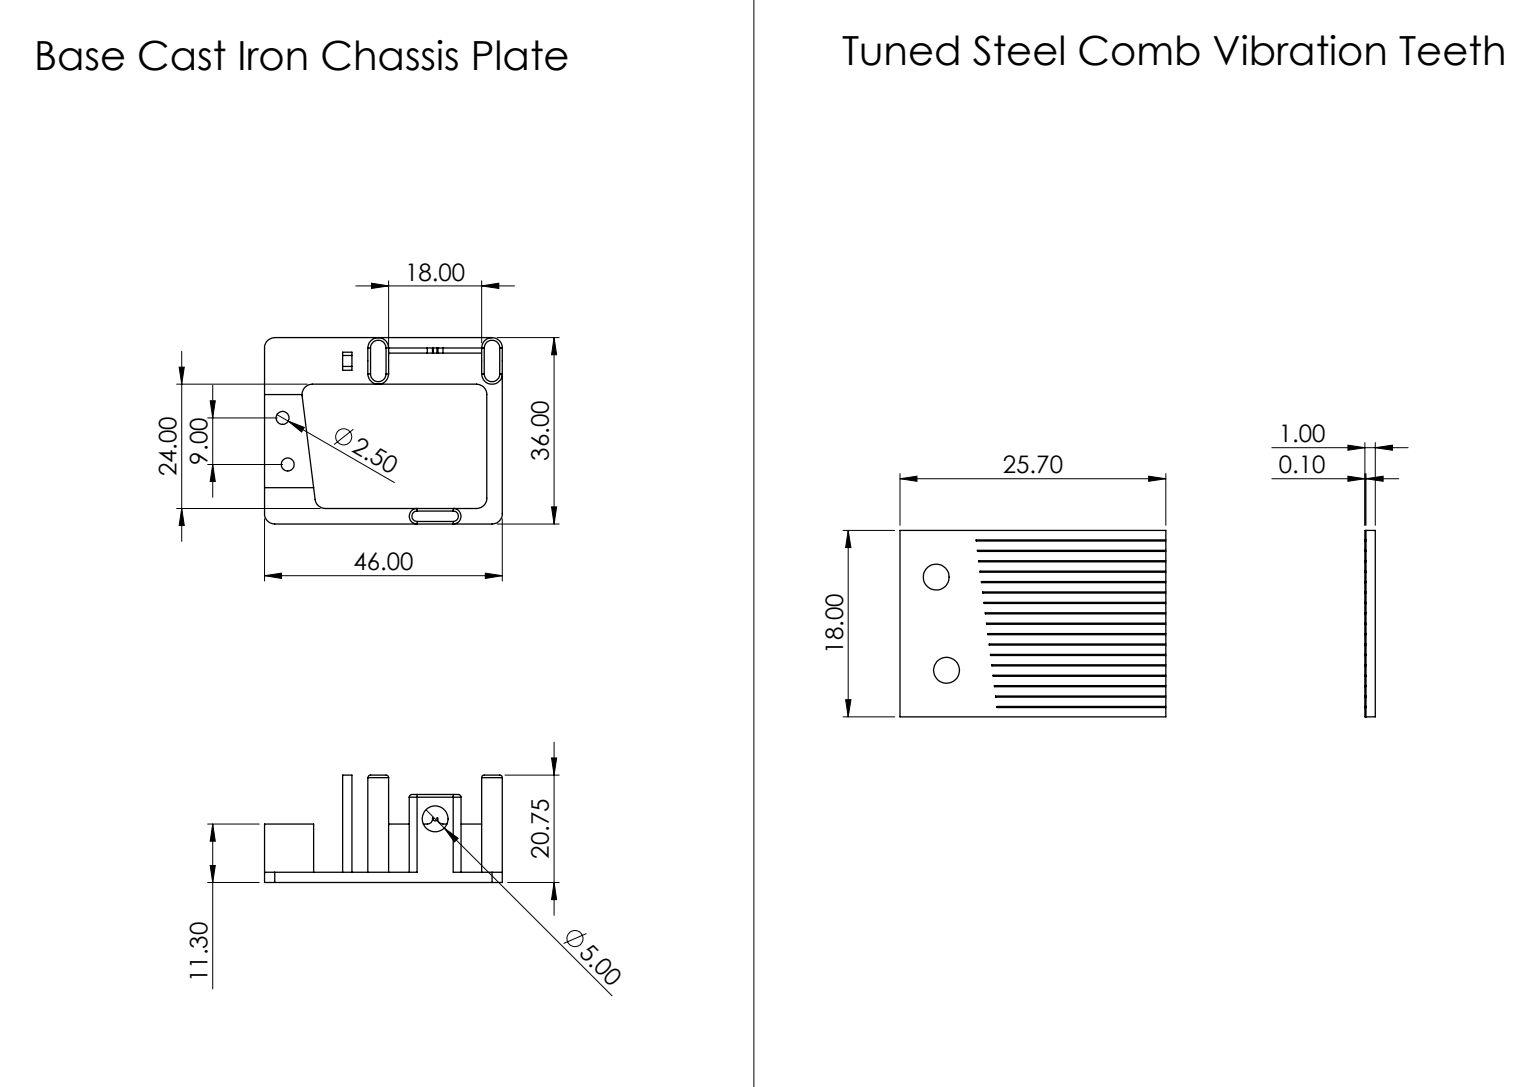
ISO-10303-21;
HEADER;
FILE_DESCRIPTION (('STEP AP214'),
    '1' );
FILE_NAME ('Base Cast Iron Chassis Plate.step',
    '2026-10-09T09:51:18',
    ( '' ),
    ( '' ),
    'SwSTEP 2.0',
    'SolidWorks 2026',
    '' );
FILE_SCHEMA (( 'AUTOMOTIVE_DESIGN' ));
ENDSEC;

DATA;
#33=EDGE_CURVE ( 'NONE', #48317, #41762, #10165, .T. ) ;
#35=DIRECTION ( 'NONE',  ( -0.000000000000000000, -1.000000000000000000, 0.000000000000000000 ) ) ;
#44=ORIENTED_EDGE ( 'NONE', *, *, #25310, .F. ) ;
#62=ADVANCED_FACE ( 'NONE', ( #10414 ), #3672, .F. ) ;
#68=CARTESIAN_POINT ( 'NONE',  ( -45.92409385541305511, -17.80920654474410370, 70.50000000000000000 ) ) ;
#96=EDGE_CURVE ( 'NONE', #20442, #47219, #874, .T. ) ;
#102=DIRECTION ( 'NONE',  ( -0.000000000000000000, -0.000000000000000000, 1.000000000000000000 ) ) ;
#112=VERTEX_POINT ( 'NONE', #24372 ) ;
#115=VERTEX_POINT ( 'NONE', #13251 ) ;
#124=CARTESIAN_POINT ( 'NONE',  ( -9.424093855413051557, -25.10920654474410441, 78.99999999999998579 ) ) ;
#130=DIRECTION ( 'NONE',  ( -1.000000000000000000, 0.000000000000000000, 0.000000000000000000 ) ) ;
#145=AXIS2_PLACEMENT_3D ( 'NONE', #27646, #26927, #38474 ) ;
#151=ORIENTED_EDGE ( 'NONE', *, *, #6962, .F. ) ;
#182=LINE ( 'NONE', #415, #745 ) ;
#226=EDGE_CURVE ( 'NONE', #34970, #8191, #23283, .T. ) ;
#271=ORIENTED_EDGE ( 'NONE', *, *, #34280, .T. ) ;
#297=ORIENTED_EDGE ( 'NONE', *, *, #9751, .F. ) ;
#323=EDGE_LOOP ( 'NONE', ( #31149, #39606, #41747, #34828, #13815, #44487, #8986, #28396, #6353, #8723, #40195, #13275, #11784, #44102 ) ) ;
#350=VECTOR ( 'NONE', #21836, 1000.000000000000000 ) ;
#374=EDGE_CURVE ( 'NONE', #44110, #112, #11065, .T. ) ;
#381=CARTESIAN_POINT ( 'NONE',  ( -45.92409385541305511, -15.80920654474410725, 70.50000000000000000 ) ) ;
#410=ORIENTED_EDGE ( 'NONE', *, *, #41877, .F. ) ;
#415=CARTESIAN_POINT ( 'NONE',  ( -26.42409385541305511, -6.859206544744110623, 63.99999999999998579 ) ) ;
#451=DIRECTION ( 'NONE',  ( 1.927470528863119542E-16, 0.000000000000000000, -1.000000000000000000 ) ) ;
#487=CARTESIAN_POINT ( 'NONE',  ( -8.424093855413060439, -6.859206544744110623, 47.99999999999998579 ) ) ;
#500=EDGE_CURVE ( 'NONE', #11264, #34652, #47330, .T. ) ;
#516=LINE ( 'NONE', #23664, #6426 ) ;
#548=AXIS2_PLACEMENT_3D ( 'NONE', #12878, #27906, #42931 ) ;
#551=ORIENTED_EDGE ( 'NONE', *, *, #1678, .F. ) ;
#568=DIRECTION ( 'NONE',  ( -0.000000000000000000, 0.000000000000000000, 1.000000000000000000 ) ) ;
#601=CARTESIAN_POINT ( 'NONE',  ( -9.424093855413051557, -27.10920654474410796, 78.99999999999998579 ) ) ;
#635=DIRECTION ( 'NONE',  ( 0.000000000000000000, 0.000000000000000000, 1.000000000000000000 ) ) ;
#645=ORIENTED_EDGE ( 'NONE', *, *, #35314, .F. ) ;
#650=ORIENTED_EDGE ( 'NONE', *, *, #25310, .T. ) ;
#652=CIRCLE ( 'NONE', #36779, 1.999999999999994893 ) ;
#667=ADVANCED_FACE ( 'NONE', ( #34162 ), #31558, .T. ) ;
#669=DIRECTION ( 'NONE',  ( -1.000000000000000000, 0.000000000000000000, 0.000000000000000000 ) ) ;
#730=VECTOR ( 'NONE', #22079, 1000.000000000000000 ) ;
#733=VERTEX_POINT ( 'NONE', #8821 ) ;
#744=VERTEX_POINT ( 'NONE', #45770 ) ;
#745=VECTOR ( 'NONE', #8958, 1000.000000000000000 ) ;
#750=AXIS2_PLACEMENT_3D ( 'NONE', #47534, #36184, #14476 ) ;
#775=CARTESIAN_POINT ( 'NONE',  ( -6.424093855413058662, -6.359206544744109735, 54.49999999999999289 ) ) ;
#823=DIRECTION ( 'NONE',  ( -0.000000000000000000, -1.000000000000000000, -0.000000000000000000 ) ) ;
#837=CARTESIAN_POINT ( 'NONE',  ( -20.92409385541305511, -10.60920654474410618, 80.49999999999998579 ) ) ;
#874=CIRCLE ( 'NONE', #39392, 1.500000000000001332 ) ;
#912=EDGE_LOOP ( 'NONE', ( #31979, #5220, #38589, #31849 ) ) ;
#948=ADVANCED_FACE ( 'NONE', ( #45222 ), #34106, .T. ) ;
#959=FACE_BOUND ( 'NONE', #40484, .T. ) ;
#966=CARTESIAN_POINT ( 'NONE',  ( -27.42409385541305511, -15.80920654474410725, 56.99999999999999289 ) ) ;
#992=ORIENTED_EDGE ( 'NONE', *, *, #27097, .F. ) ;
#1026=CARTESIAN_POINT ( 'NONE',  ( -50.42409385541304800, -27.10920654474410796, 79.99999999999998579 ) ) ;
#1037=EDGE_CURVE ( 'NONE', #115, #47219, #27621, .T. ) ;
#1056=ADVANCED_FACE ( 'NONE', ( #4331 ), #19586, .F. ) ;
#1102=ORIENTED_EDGE ( 'NONE', *, *, #46888, .F. ) ;
#1148=ORIENTED_EDGE ( 'NONE', *, *, #13070, .T. ) ;
#1157=CARTESIAN_POINT ( 'NONE',  ( -50.42509385541305988, -6.359206544744109735, 51.54999999999998295 ) ) ;
#1179=VERTEX_POINT ( 'NONE', #43465 ) ;
#1180=CARTESIAN_POINT ( 'NONE',  ( -13.92409385541305511, -10.60920654474410618, 80.49999999999998579 ) ) ;
#1181=DIRECTION ( 'NONE',  ( -1.000000000000000000, 0.000000000000000000, 0.000000000000000000 ) ) ;
#1236=LINE ( 'NONE', #31282, #23232 ) ;
#1248=DIRECTION ( 'NONE',  ( 1.000000000000000000, 0.000000000000000000, -3.652049423109068320E-16 ) ) ;
#1253=LINE ( 'NONE', #27121, #32144 ) ;
#1275=ORIENTED_EDGE ( 'NONE', *, *, #35978, .T. ) ;
#1284=EDGE_CURVE ( 'NONE', #37234, #30602, #37046, .T. ) ;
#1287=DIRECTION ( 'NONE',  ( -0.000000000000000000, -1.000000000000000000, -0.000000000000000000 ) ) ;
#1300=CARTESIAN_POINT ( 'NONE',  ( -48.42409385541304800, -25.10920654474410441, 45.99999999999998579 ) ) ;
#1331=CIRCLE ( 'NONE', #45403, 1.250000000000001110 ) ;
#1333=CARTESIAN_POINT ( 'NONE',  ( -50.42409385541304800, -25.10920654474410441, 79.99999999999998579 ) ) ;
#1338=VECTOR ( 'NONE', #13076, 1000.000000000000000 ) ;
#1350=ADVANCED_FACE ( 'NONE', ( #23234 ), #45656, .F. ) ;
#1363=EDGE_LOOP ( 'NONE', ( #16129, #27063 ) ) ;
#1371=CARTESIAN_POINT ( 'NONE',  ( -29.92409385541305156, -6.859206544744110623, 52.99999999999997158 ) ) ;
#1373=VECTOR ( 'NONE', #12491, 1000.000000000000000 ) ;
#1377=ADVANCED_FACE ( 'NONE', ( #37744 ), #4039, .F. ) ;
#1418=CARTESIAN_POINT ( 'NONE',  ( -4.924093855413050669, -6.859206544744110623, 47.99999999999998579 ) ) ;
#1424=CYLINDRICAL_SURFACE ( 'NONE', #27500, 0.5000000000000004441 ) ;
#1428=CARTESIAN_POINT ( 'NONE',  ( -27.42409385541305511, -25.10920654474410441, 63.99999999999998579 ) ) ;
#1443=CARTESIAN_POINT ( 'NONE',  ( -6.424093855413058662, -6.859206544744110623, 52.99999999999998579 ) ) ;
#1445=VECTOR ( 'NONE', #43605, 1000.000000000000000 ) ;
#1467=ADVANCED_FACE ( 'NONE', ( #5493 ), #1787, .T. ) ;
#1472=DIRECTION ( 'NONE',  ( 0.000000000000000000, 0.000000000000000000, 1.000000000000000000 ) ) ;
#1541=CARTESIAN_POINT ( 'NONE',  ( -28.42409385541305511, -6.859206544744110623, 47.99999999999997868 ) ) ;
#1543=DIRECTION ( 'NONE',  ( -9.637352644315596475E-17, 0.000000000000000000, -1.000000000000000000 ) ) ;
#1549=CARTESIAN_POINT ( 'NONE',  ( -17.90106345612152694, -14.65920654474411045, 47.99999999999998579 ) ) ;
#1552=CARTESIAN_POINT ( 'NONE',  ( -33.52409385541305653, -8.109206544744111511, 51.54999999999998295 ) ) ;
#1633=CIRCLE ( 'NONE', #34671, 1.250000000000001110 ) ;
#1645=VERTEX_POINT ( 'NONE', #44857 ) ;
#1659=ORIENTED_EDGE ( 'NONE', *, *, #39608, .F. ) ;
#1668=EDGE_LOOP ( 'NONE', ( #31560, #32124, #35953, #44439 ) ) ;
#1678=EDGE_CURVE ( 'NONE', #36016, #25288, #21372, .T. ) ;
#1713=EDGE_CURVE ( 'NONE', #32365, #12722, #516, .T. ) ;
#1728=EDGE_CURVE ( 'NONE', #2748, #17620, #30813, .T. ) ;
#1738=CARTESIAN_POINT ( 'NONE',  ( -7.924093855413094190, -6.859206544744110623, 64.00000000000002842 ) ) ;
#1764=FACE_OUTER_BOUND ( 'NONE', #6246, .T. ) ;
#1787=CYLINDRICAL_SURFACE ( 'NONE', #19009, 1.500000000000001332 ) ;
#1796=ORIENTED_EDGE ( 'NONE', *, *, #30506, .T. ) ;
#1809=ORIENTED_EDGE ( 'NONE', *, *, #35759, .T. ) ;
#1836=VERTEX_POINT ( 'NONE', #39874 ) ;
#1838=CARTESIAN_POINT ( 'NONE',  ( -20.92409385541305511, -10.10920654474410618, 79.49999999999998579 ) ) ;
#1848=DIRECTION ( 'NONE',  ( 1.000000000000000000, 0.000000000000000000, 0.000000000000000000 ) ) ;
#1855=DIRECTION ( 'NONE',  ( -0.000000000000000000, -0.000000000000000000, -1.000000000000000000 ) ) ;
#1860=ORIENTED_EDGE ( 'NONE', *, *, #23584, .T. ) ;
#1928=ORIENTED_EDGE ( 'NONE', *, *, #8269, .F. ) ;
#1937=EDGE_CURVE ( 'NONE', #47219, #16341, #7128, .T. ) ;
#1967=PLANE ( 'NONE',  #12522 ) ;
#2011=AXIS2_PLACEMENT_3D ( 'NONE', #15786, #26648, #7705 ) ;
#2020=PLANE ( 'NONE',  #18780 ) ;
#2057=CIRCLE ( 'NONE', #38202, 2.000000000000008882 ) ;
#2088=CARTESIAN_POINT ( 'NONE',  ( -27.42409385541305511, -25.10920654474410441, 78.99999999999998579 ) ) ;
#2100=VERTEX_POINT ( 'NONE', #11302 ) ;
#2103=EDGE_CURVE ( 'NONE', #46918, #14429, #23355, .T. ) ;
#2112=ADVANCED_FACE ( 'NONE', ( #7867 ), #22887, .T. ) ;
#2115=DIRECTION ( 'NONE',  ( -0.000000000000000000, -1.000000000000000000, -0.000000000000000000 ) ) ;
#2123=DIRECTION ( 'NONE',  ( 0.000000000000000000, -0.000000000000000000, 1.000000000000000000 ) ) ;
#2158=AXIS2_PLACEMENT_3D ( 'NONE', #31094, #42182, #35506 ) ;
#2182=ORIENTED_EDGE ( 'NONE', *, *, #13017, .F. ) ;
#2215=CIRCLE ( 'NONE', #14755, 1.000000000000000888 ) ;
#2221=DIRECTION ( 'NONE',  ( 0.000000000000000000, 0.000000000000000000, -1.000000000000000000 ) ) ;
#2247=( GEOMETRIC_REPRESENTATION_CONTEXT ( 3 ) GLOBAL_UNCERTAINTY_ASSIGNED_CONTEXT ( ( #43031 ) ) GLOBAL_UNIT_ASSIGNED_CONTEXT ( ( #15533, #27609, #34253 ) ) REPRESENTATION_CONTEXT ( 'NONE', 'WORKASPACE' ) );
#2252=LINE ( 'NONE', #10130, #2355 ) ;
#2276=CARTESIAN_POINT ( 'NONE',  ( -9.424093855413051557, -27.10920654474410796, 77.00000000000000000 ) ) ;
#2283=DIRECTION ( 'NONE',  ( 0.000000000000000000, 0.000000000000000000, 1.000000000000000000 ) ) ;
#2306=EDGE_CURVE ( 'NONE', #733, #9420, #33312, .T. ) ;
#2310=CYLINDRICAL_SURFACE ( 'NONE', #27292, 2.000000000000001776 ) ;
#2314=ORIENTED_EDGE ( 'NONE', *, *, #36771, .F. ) ;
#2334=ADVANCED_FACE ( 'NONE', ( #7998 ), #8714, .T. ) ;
#2355=VECTOR ( 'NONE', #21692, 1000.000000000000000 ) ;
#2371=CARTESIAN_POINT ( 'NONE',  ( -28.42409385541305511, -6.859206544744110623, 52.99999999999997158 ) ) ;
#2376=EDGE_CURVE ( 'NONE', #38493, #28218, #38231, .T. ) ;
#2394=EDGE_CURVE ( 'NONE', #45181, #19972, #31347, .T. ) ;
#2399=CARTESIAN_POINT ( 'NONE',  ( -26.42409385541305511, -25.10920654474410441, 63.99999999999998579 ) ) ;
#2409=CARTESIAN_POINT ( 'NONE',  ( -14.92409385541305333, -14.80920654474410725, 45.99899999999998101 ) ) ;
#2411=DIRECTION ( 'NONE',  ( -1.000000000000000000, -0.000000000000000000, -0.000000000000000000 ) ) ;
#2415=ORIENTED_EDGE ( 'NONE', *, *, #29630, .F. ) ;
#2465=ORIENTED_EDGE ( 'NONE', *, *, #32444, .T. ) ;
#2490=AXIS2_PLACEMENT_3D ( 'NONE', #46219, #42772, #12478 ) ;
#2505=LINE ( 'NONE', #9900, #9737 ) ;
#2511=DIRECTION ( 'NONE',  ( -0.000000000000000000, -1.000000000000000000, -0.000000000000000000 ) ) ;
#2528=CARTESIAN_POINT ( 'NONE',  ( -30.42409385541305156, -25.10920654474410441, 63.99999999999998579 ) ) ;
#2535=EDGE_CURVE ( 'NONE', #4116, #25391, #4552, .T. ) ;
#2584=CYLINDRICAL_SURFACE ( 'NONE', #9338, 1.000000000000000888 ) ;
#2597=PLANE ( 'NONE',  #44083 ) ;
#2600=EDGE_CURVE ( 'NONE', #28218, #43409, #29728, .T. ) ;
#2616=CIRCLE ( 'NONE', #42741, 0.5000000000000004441 ) ;
#2631=VERTEX_POINT ( 'NONE', #22447 ) ;
#2645=DIRECTION ( 'NONE',  ( -1.000000000000000000, 0.000000000000000000, 0.000000000000000000 ) ) ;
#2671=CARTESIAN_POINT ( 'NONE',  ( -26.42409385541305511, -25.10920654474410441, 48.99999999999997868 ) ) ;
#2712=ORIENTED_EDGE ( 'NONE', *, *, #10175, .T. ) ;
#2722=DIRECTION ( 'NONE',  ( 0.000000000000000000, 0.000000000000000000, -1.000000000000000000 ) ) ;
#2743=VECTOR ( 'NONE', #5325, 1000.000000000000000 ) ;
#2748=VERTEX_POINT ( 'NONE', #27598 ) ;
#2752=VERTEX_POINT ( 'NONE', #775 ) ;
#2784=EDGE_LOOP ( 'NONE', ( #33088, #44144, #32827, #44767 ) ) ;
#2785=DIRECTION ( 'NONE',  ( -1.000000000000000000, 0.000000000000000000, -0.000000000000000000 ) ) ;
#2830=FACE_OUTER_BOUND ( 'NONE', #323, .T. ) ;
#2839=EDGE_CURVE ( 'NONE', #21252, #31120, #13526, .T. ) ;
#2843=LINE ( 'NONE', #18096, #44954 ) ;
#2855=CARTESIAN_POINT ( 'NONE',  ( -20.92409385541305511, -10.60920654474410618, 81.49999999999998579 ) ) ;
#2906=VECTOR ( 'NONE', #39292, 1000.000000000000000 ) ;
#2941=DIRECTION ( 'NONE',  ( 1.000000000000000000, -0.000000000000000000, 2.168404344971008375E-16 ) ) ;
#2947=DIRECTION ( 'NONE',  ( 0.000000000000000000, 0.000000000000000000, 1.000000000000000000 ) ) ;
#2959=CARTESIAN_POINT ( 'NONE',  ( -8.424093855413067544, -8.109206544744111511, 50.49999999999999289 ) ) ;
#2982=AXIS2_PLACEMENT_3D ( 'NONE', #26974, #23958, #28376 ) ;
#2993=DIRECTION ( 'NONE',  ( 0.000000000000000000, 0.000000000000000000, 1.000000000000000000 ) ) ;
#3018=STYLED_ITEM ( 'NONE', ( #7702 ), #48569 ) ;
#3046=AXIS2_PLACEMENT_3D ( 'NONE', #41887, #41639, #15267 ) ;
#3084=DIRECTION ( 'NONE',  ( 1.000000000000000000, -0.000000000000000000, 0.000000000000000000 ) ) ;
#3088=DIRECTION ( 'NONE',  ( -0.000000000000000000, -1.000000000000000000, -0.000000000000000000 ) ) ;
#3140=DIRECTION ( 'NONE',  ( 0.000000000000000000, 0.000000000000000000, 1.000000000000000000 ) ) ;
#3190=LINE ( 'NONE', #29057, #27320 ) ;
#3197=ORIENTED_EDGE ( 'NONE', *, *, #37500, .F. ) ;
#3204=DIRECTION ( 'NONE',  ( -1.000000000000000000, 0.000000000000000000, 0.000000000000000000 ) ) ;
#3206=AXIS2_PLACEMENT_3D ( 'NONE', #13898, #33092, #28940 ) ;
#3226=AXIS2_PLACEMENT_3D ( 'NONE', #40066, #17639, #22564 ) ;
#3273=EDGE_CURVE ( 'NONE', #37009, #33767, #33383, .T. ) ;
#3289=ORIENTED_EDGE ( 'NONE', *, *, #27097, .T. ) ;
#3293=LINE ( 'NONE', #30142, #44747 ) ;
#3328=EDGE_CURVE ( 'NONE', #14429, #38493, #11008, .T. ) ;
#3335=EDGE_CURVE ( 'NONE', #34669, #48317, #22329, .T. ) ;
#3347=ORIENTED_EDGE ( 'NONE', *, *, #21881, .T. ) ;
#3378=DIRECTION ( 'NONE',  ( -0.000000000000000000, 1.000000000000000000, -0.000000000000000000 ) ) ;
#3383=VERTEX_POINT ( 'NONE', #41785 ) ;
#3449=TOROIDAL_SURFACE ( 'NONE', #16811, 1.000000000000001332, 0.5000000000000000000 ) ;
#3536=ADVANCED_FACE ( 'NONE', ( #46943 ), #13185, .T. ) ;
#3538=ORIENTED_EDGE ( 'NONE', *, *, #32461, .F. ) ;
#3542=ORIENTED_EDGE ( 'NONE', *, *, #35910, .T. ) ;
#3550=CARTESIAN_POINT ( 'NONE',  ( -46.92409385541305511, -17.80920654474410370, 61.49999999999999289 ) ) ;
#3580=EDGE_CURVE ( 'NONE', #48493, #10239, #43746, .T. ) ;
#3584=LINE ( 'NONE', #19098, #27397 ) ;
#3590=VECTOR ( 'NONE', #43857, 1000.000000000000000 ) ;
#3619=EDGE_CURVE ( 'NONE', #26610, #45033, #14381, .T. ) ;
#3623=ORIENTED_EDGE ( 'NONE', *, *, #33387, .T. ) ;
#3647=VERTEX_POINT ( 'NONE', #44470 ) ;
#3672=PLANE ( 'NONE',  #47239 ) ;
#3701=AXIS2_PLACEMENT_3D ( 'NONE', #45812, #38147, #38389 ) ;
#3721=CARTESIAN_POINT ( 'NONE',  ( -46.92409385541305511, -15.80920654474410725, 62.75000000000000000 ) ) ;
#3745=FACE_OUTER_BOUND ( 'NONE', #38121, .T. ) ;
#3769=DIRECTION ( 'NONE',  ( 1.000000000000000000, -0.000000000000000000, -2.406186529621654511E-16 ) ) ;
#3773=CIRCLE ( 'NONE', #47805, 2.000000000000001776 ) ;
#3781=ADVANCED_FACE ( 'NONE', ( #33345, #38029 ), #44972, .F. ) ;
#3803=ORIENTED_EDGE ( 'NONE', *, *, #21440, .F. ) ;
#3822=CIRCLE ( 'NONE', #46286, 1.500000000000001332 ) ;
#3823=DIRECTION ( 'NONE',  ( 0.000000000000000000, 0.000000000000000000, -1.000000000000000000 ) ) ;
#3826=EDGE_CURVE ( 'NONE', #34652, #19690, #19421, .T. ) ;
#3842=VERTEX_POINT ( 'NONE', #46659 ) ;
#3853=CIRCLE ( 'NONE', #36815, 0.5000000000000004441 ) ;
#3854=AXIS2_PLACEMENT_3D ( 'NONE', #42661, #9160, #4740 ) ;
#3895=VERTEX_POINT ( 'NONE', #16097 ) ;
#3906=ORIENTED_EDGE ( 'NONE', *, *, #21440, .T. ) ;
#3921=DIRECTION ( 'NONE',  ( -1.000000000000000000, 0.000000000000000000, -2.181982678098338148E-16 ) ) ;
#3936=CARTESIAN_POINT ( 'NONE',  ( -15.92409385541305333, -14.80920654474410547, 47.99999999999998579 ) ) ;
#3944=ORIENTED_EDGE ( 'NONE', *, *, #12913, .T. ) ;
#3947=EDGE_CURVE ( 'NONE', #37009, #3647, #28896, .T. ) ;
#3950=AXIS2_PLACEMENT_3D ( 'NONE', #4500, #568, #19520 ) ;
#3959=CIRCLE ( 'NONE', #7127, 0.5000000000000004441 ) ;
#3983=ORIENTED_EDGE ( 'NONE', *, *, #3619, .T. ) ;
#3987=ORIENTED_EDGE ( 'NONE', *, *, #21722, .F. ) ;
#3991=CARTESIAN_POINT ( 'NONE',  ( -27.42409385541305511, -10.60920654474410618, 79.49999999999998579 ) ) ;
#4010=ORIENTED_EDGE ( 'NONE', *, *, #2376, .F. ) ;
#4039=PLANE ( 'NONE',  #145 ) ;
#4096=AXIS2_PLACEMENT_3D ( 'NONE', #18266, #14315, #33271 ) ;
#4114=ORIENTED_EDGE ( 'NONE', *, *, #28826, .F. ) ;
#4116=VERTEX_POINT ( 'NONE', #26420 ) ;
#4125=VERTEX_POINT ( 'NONE', #40699 ) ;
#4154=DIRECTION ( 'NONE',  ( 0.000000000000000000, 0.000000000000000000, -1.000000000000000000 ) ) ;
#4187=ORIENTED_EDGE ( 'NONE', *, *, #31377, .F. ) ;
#4205=EDGE_CURVE ( 'NONE', #39884, #41525, #35926, .T. ) ;
#4223=DIRECTION ( 'NONE',  ( -1.000000000000000000, 0.000000000000000000, 0.000000000000000000 ) ) ;
#4232=LINE ( 'NONE', #33756, #6022 ) ;
#4235=EDGE_CURVE ( 'NONE', #31166, #20442, #16532, .T. ) ;
#4242=SURFACE_SIDE_STYLE ('',( #23437 ) ) ;
#4270=CARTESIAN_POINT ( 'NONE',  ( -50.42509385541305988, -8.109206544744111511, 51.54999999999998295 ) ) ;
#4280=CIRCLE ( 'NONE', #40436, 1.250000000000007994 ) ;
#4300=CARTESIAN_POINT ( 'NONE',  ( -33.52409385541305653, -8.109206544744111511, 50.49999999999998579 ) ) ;
#4312=EDGE_CURVE ( 'NONE', #2748, #38065, #32301, .T. ) ;
#4331=FACE_OUTER_BOUND ( 'NONE', #30439, .T. ) ;
#4362=CYLINDRICAL_SURFACE ( 'NONE', #14996, 0.3999999999999975797 ) ;
#4377=ORIENTED_EDGE ( 'NONE', *, *, #21519, .T. ) ;
#4379=FACE_OUTER_BOUND ( 'NONE', #37075, .T. ) ;
#4393=DIRECTION ( 'NONE',  ( 0.000000000000000000, 1.000000000000000000, -0.000000000000000000 ) ) ;
#4395=ORIENTED_EDGE ( 'NONE', *, *, #7324, .T. ) ;
#4409=AXIS2_PLACEMENT_3D ( 'NONE', #10539, #6602, #14670 ) ;
#4449=EDGE_LOOP ( 'NONE', ( #31051, #29171, #21182, #15665 ) ) ;
#4484=CARTESIAN_POINT ( 'NONE',  ( -33.52409385541305653, -8.109206544744111511, 49.44999999999998863 ) ) ;
#4500=CARTESIAN_POINT ( 'NONE',  ( -26.92409385541305511, -6.859206544744110623, 63.99999999999998579 ) ) ;
#4510=CIRCLE ( 'NONE', #43861, 2.000000000000001776 ) ;
#4520=AXIS2_PLACEMENT_3D ( 'NONE', #48634, #11453, #37794 ) ;
#4552=CIRCLE ( 'NONE', #26567, 1.250000000000007994 ) ;
#4560=ORIENTED_EDGE ( 'NONE', *, *, #374, .T. ) ;
#4583=DIRECTION ( 'NONE',  ( -1.000000000000000000, 0.000000000000000000, 0.000000000000000000 ) ) ;
#4593=CIRCLE ( 'NONE', #10879, 0.5000000000000004441 ) ;
#4636=CARTESIAN_POINT ( 'NONE',  ( -27.42409385541305511, -6.359206544744109735, 63.99999999999998579 ) ) ;
#4647=EDGE_LOOP ( 'NONE', ( #16547, #20714, #20087, #44 ) ) ;
#4663=ORIENTED_EDGE ( 'NONE', *, *, #17376, .T. ) ;
#4664=DIRECTION ( 'NONE',  ( 2.081668171172170091E-15, -0.000000000000000000, -1.000000000000000000 ) ) ;
#4687=VERTEX_POINT ( 'NONE', #26004 ) ;
#4740=DIRECTION ( 'NONE',  ( 0.000000000000000000, 0.000000000000000000, 1.000000000000000000 ) ) ;
#4750=DIRECTION ( 'NONE',  ( 1.000000000000000000, -0.000000000000000000, 2.081668171172170091E-15 ) ) ;
#4760=LINE ( 'NONE', #8705, #37634 ) ;
#4768=ORIENTED_EDGE ( 'NONE', *, *, #10574, .F. ) ;
#4788=DIRECTION ( 'NONE',  ( -0.000000000000000000, -1.000000000000000000, -0.000000000000000000 ) ) ;
#4794=AXIS2_PLACEMENT_3D ( 'NONE', #23904, #35203, #1472 ) ;
#4808=LINE ( 'NONE', #1333, #4834 ) ;
#4818=ORIENTED_EDGE ( 'NONE', *, *, #21563, .T. ) ;
#4834=VECTOR ( 'NONE', #19832, 1000.000000000000000 ) ;
#4931=EDGE_CURVE ( 'NONE', #7384, #17465, #43953, .T. ) ;
#4953=LINE ( 'NONE', #35931, #31027 ) ;
#4984=VERTEX_POINT ( 'NONE', #6015 ) ;
#5031=DIRECTION ( 'NONE',  ( 0.000000000000000000, 1.000000000000000000, -0.000000000000000000 ) ) ;
#5034=CYLINDRICAL_SURFACE ( 'NONE', #44890, 2.000000000000001776 ) ;
#5053=ADVANCED_FACE ( 'NONE', ( #10927 ), #11405, .F. ) ;
#5070=CARTESIAN_POINT ( 'NONE',  ( -42.07024770156689897, -25.10920654474410441, 65.83076923076922071 ) ) ;
#5074=VERTEX_POINT ( 'NONE', #48588 ) ;
#5088=DIRECTION ( 'NONE',  ( 0.000000000000000000, 0.000000000000000000, 1.000000000000000000 ) ) ;
#5104=LINE ( 'NONE', #45506, #26905 ) ;
#5112=CARTESIAN_POINT ( 'NONE',  ( -8.424093855413067544, -6.859206544744110623, 50.49999999999999289 ) ) ;
#5140=FACE_OUTER_BOUND ( 'NONE', #32706, .T. ) ;
#5167=DIRECTION ( 'NONE',  ( -0.000000000000000000, -1.000000000000000000, -0.000000000000000000 ) ) ;
#5176=EDGE_CURVE ( 'NONE', #1179, #30092, #29680, .T. ) ;
#5182=ORIENTED_EDGE ( 'NONE', *, *, #48088, .F. ) ;
#5202=DIRECTION ( 'NONE',  ( 0.000000000000000000, 0.000000000000000000, 1.000000000000000000 ) ) ;
#5216=VERTEX_POINT ( 'NONE', #12855 ) ;
#5220=ORIENTED_EDGE ( 'NONE', *, *, #31630, .F. ) ;
#5228=DIRECTION ( 'NONE',  ( 2.168404344971008375E-16, -0.000000000000000000, -1.000000000000000000 ) ) ;
#5233=CARTESIAN_POINT ( 'NONE',  ( -27.42409385541305511, -6.359206544744109735, 63.99999999999998579 ) ) ;
#5263=AXIS2_PLACEMENT_3D ( 'NONE', #19439, #12535, #41859 ) ;
#5276=ORIENTED_EDGE ( 'NONE', *, *, #36050, .F. ) ;
#5315=DIRECTION ( 'NONE',  ( 1.000000000000000000, 0.000000000000000000, 8.260587980841940012E-17 ) ) ;
#5325=DIRECTION ( 'NONE',  ( 1.000000000000000000, -0.000000000000000000, -2.406186529621654511E-16 ) ) ;
#5342=VERTEX_POINT ( 'NONE', #24916 ) ;
#5356=DIRECTION ( 'NONE',  ( -0.000000000000000000, -1.000000000000000000, -0.000000000000000000 ) ) ;
#5358=EDGE_LOOP ( 'NONE', ( #3347, #22271, #271, #46767 ) ) ;
#5359=DIRECTION ( 'NONE',  ( 0.000000000000000000, 0.000000000000000000, -1.000000000000000000 ) ) ;
#5360=VECTOR ( 'NONE', #38478, 1000.000000000000000 ) ;
#5381=ORIENTED_EDGE ( 'NONE', *, *, #40240, .F. ) ;
#5388=CARTESIAN_POINT ( 'NONE',  ( -4.424093855413053333, -6.859206544744110623, 63.99999999999998579 ) ) ;
#5400=AXIS2_PLACEMENT_3D ( 'NONE', #40482, #21309, #10226 ) ;
#5416=ORIENTED_EDGE ( 'NONE', *, *, #34630, .F. ) ;
#5464=VERTEX_POINT ( 'NONE', #30268 ) ;
#5472=CIRCLE ( 'NONE', #32952, 1.250000000000001110 ) ;
#5482=ORIENTED_EDGE ( 'NONE', *, *, #9948, .T. ) ;
#5493=FACE_OUTER_BOUND ( 'NONE', #27867, .T. ) ;
#5513=AXIS2_PLACEMENT_3D ( 'NONE', #28993, #2411, #43548 ) ;
#5528=VECTOR ( 'NONE', #32490, 1000.000000000000000 ) ;
#5536=AXIS2_PLACEMENT_3D ( 'NONE', #39076, #23342, #5359 ) ;
#5537=FACE_OUTER_BOUND ( 'NONE', #16531, .T. ) ;
#5577=CARTESIAN_POINT ( 'NONE',  ( -16.92409385541305511, -14.80920654474410547, 47.99999999999998579 ) ) ;
#5628=ORIENTED_EDGE ( 'NONE', *, *, #14146, .T. ) ;
#5693=CARTESIAN_POINT ( 'NONE',  ( -19.92409385541305511, -14.80920654474410725, 81.99999999999998579 ) ) ;
#5708=CARTESIAN_POINT ( 'NONE',  ( -28.42409385541305511, -6.859206544744110623, 54.49999999999997158 ) ) ;
#5709=DIRECTION ( 'NONE',  ( -1.000000000000000000, 0.000000000000000000, 0.000000000000000000 ) ) ;
#5713=EDGE_LOOP ( 'NONE', ( #17413, #19574, #44445, #44070, #28697, #28326, #10093, #10707 ) ) ;
#5769=ORIENTED_EDGE ( 'NONE', *, *, #29800, .F. ) ;
#5783=DIRECTION ( 'NONE',  ( 0.000000000000000000, 0.000000000000000000, 1.000000000000000000 ) ) ;
#5784=ORIENTED_EDGE ( 'NONE', *, *, #14022, .F. ) ;
#5801=DIRECTION ( 'NONE',  ( 1.000000000000000000, -0.000000000000000000, 0.000000000000000000 ) ) ;
#5802=AXIS2_PLACEMENT_3D ( 'NONE', #20502, #16782, #35016 ) ;
#5808=ORIENTED_EDGE ( 'NONE', *, *, #17494, .T. ) ;
#5811=ORIENTED_EDGE ( 'NONE', *, *, #21811, .F. ) ;
#5835=LINE ( 'NONE', #20846, #38331 ) ;
#5856=ORIENTED_EDGE ( 'NONE', *, *, #13548, .T. ) ;
#5877=ADVANCED_FACE ( 'NONE', ( #26752 ), #41772, .T. ) ;
#5881=CARTESIAN_POINT ( 'NONE',  ( -41.15852941833841783, -25.10920654474410441, 56.99999999999997868 ) ) ;
#5890=EDGE_CURVE ( 'NONE', #2631, #18891, #10070, .T. ) ;
#5919=LINE ( 'NONE', #21660, #48472 ) ;
#5923=PLANE ( 'NONE',  #44000 ) ;
#5936=DIRECTION ( 'NONE',  ( 0.000000000000000000, 0.000000000000000000, 1.000000000000000000 ) ) ;
#5959=CYLINDRICAL_SURFACE ( 'NONE', #2982, 2.000000000000001776 ) ;
#5967=CARTESIAN_POINT ( 'NONE',  ( -27.42409385541305156, -15.80920654474410725, 74.99999999999998579 ) ) ;
#5970=DIRECTION ( 'NONE',  ( 0.000000000000000000, 0.000000000000000000, 1.000000000000000000 ) ) ;
#5984=CYLINDRICAL_SURFACE ( 'NONE', #23540, 1.250000000000001110 ) ;
#6004=DIRECTION ( 'NONE',  ( 0.000000000000000000, 0.000000000000000000, 1.000000000000000000 ) ) ;
#6011=DIRECTION ( 'NONE',  ( 1.000000000000000000, -0.000000000000000000, -2.406186529621654511E-16 ) ) ;
#6014=DIRECTION ( 'NONE',  ( -0.000000000000000000, -1.000000000000000000, -0.000000000000000000 ) ) ;
#6015=CARTESIAN_POINT ( 'NONE',  ( -17.92409385541305511, -14.80920654474410725, 47.99999999999998579 ) ) ;
#6022=VECTOR ( 'NONE', #22957, 1000.000000000000000 ) ;
#6034=ORIENTED_EDGE ( 'NONE', *, *, #1284, .F. ) ;
#6061=ORIENTED_EDGE ( 'NONE', *, *, #46657, .F. ) ;
#6100=LINE ( 'NONE', #2409, #28203 ) ;
#6125=VECTOR ( 'NONE', #33862, 1000.000000000000000 ) ;
#6128=AXIS2_PLACEMENT_3D ( 'NONE', #1738, #27590, #16004 ) ;
#6155=CARTESIAN_POINT ( 'NONE',  ( -26.42409385541305511, -15.80920654474410725, 47.99999999999997868 ) ) ;
#6164=AXIS2_PLACEMENT_3D ( 'NONE', #3991, #15282, #8178 ) ;
#6165=PLANE ( 'NONE',  #750 ) ;
#6196=DIRECTION ( 'NONE',  ( 0.000000000000000000, 1.000000000000000000, -0.000000000000000000 ) ) ;
#6197=ORIENTED_EDGE ( 'NONE', *, *, #34630, .T. ) ;
#6199=EDGE_CURVE ( 'NONE', #4984, #8191, #4593, .T. ) ;
#6246=EDGE_LOOP ( 'NONE', ( #7899, #31176, #19146, #15541 ) ) ;
#6247=ORIENTED_EDGE ( 'NONE', *, *, #20266, .F. ) ;
#6258=DIRECTION ( 'NONE',  ( 1.000000000000000000, 0.000000000000000000, 1.927470528863119295E-16 ) ) ;
#6259=ORIENTED_EDGE ( 'NONE', *, *, #6547, .F. ) ;
#6282=FACE_OUTER_BOUND ( 'NONE', #15412, .T. ) ;
#6314=DIRECTION ( 'NONE',  ( -0.000000000000000000, -1.000000000000000000, 0.000000000000000000 ) ) ;
#6315=DIRECTION ( 'NONE',  ( -0.000000000000000000, -1.000000000000000000, 0.000000000000000000 ) ) ;
#6329=ADVANCED_FACE ( 'NONE', ( #8647 ), #27102, .T. ) ;
#6349=ADVANCED_FACE ( 'NONE', ( #45512 ), #29998, .F. ) ;
#6353=ORIENTED_EDGE ( 'NONE', *, *, #39944, .F. ) ;
#6356=VECTOR ( 'NONE', #22805, 1000.000000000000000 ) ;
#6379=EDGE_CURVE ( 'NONE', #27994, #8183, #42347, .T. ) ;
#6389=CYLINDRICAL_SURFACE ( 'NONE', #20548, 2.500000000000000444 ) ;
#6392=EDGE_LOOP ( 'NONE', ( #42363, #3987, #33703, #38748, #31786, #15695, #7014, #12592 ) ) ;
#6398=CARTESIAN_POINT ( 'NONE',  ( -45.92409385541305511, -15.80920654474410725, 69.24999999999998579 ) ) ;
#6400=ORIENTED_EDGE ( 'NONE', *, *, #21745, .F. ) ;
#6411=CIRCLE ( 'NONE', #21353, 1.250000000000001110 ) ;
#6426=VECTOR ( 'NONE', #30329, 1000.000000000000000 ) ;
#6439=CIRCLE ( 'NONE', #8808, 2.000000000000001776 ) ;
#6501=CARTESIAN_POINT ( 'NONE',  ( -35.32409385541306079, -2.423472813913224222, 52.29999999999998295 ) ) ;
#6547=EDGE_CURVE ( 'NONE', #48469, #12722, #3822, .T. ) ;
#6602=DIRECTION ( 'NONE',  ( -0.000000000000000000, 1.000000000000000000, -0.000000000000000000 ) ) ;
#6609=CARTESIAN_POINT ( 'NONE',  ( -50.42509385541305988, -6.359206544744109735, 49.44999999999998863 ) ) ;
#6613=EDGE_CURVE ( 'NONE', #5216, #48283, #3584, .T. ) ;
#6639=ORIENTED_EDGE ( 'NONE', *, *, #34501, .F. ) ;
#6643=DIRECTION ( 'NONE',  ( -0.000000000000000000, -1.000000000000000000, -0.000000000000000000 ) ) ;
#6725=DIRECTION ( 'NONE',  ( 0.000000000000000000, 0.000000000000000000, 1.000000000000000000 ) ) ;
#6768=AXIS2_PLACEMENT_3D ( 'NONE', #25204, #32812, #43441 ) ;
#6790=CIRCLE ( 'NONE', #18580, 0.5000000000000004441 ) ;
#6822=ORIENTED_EDGE ( 'NONE', *, *, #12122, .F. ) ;
#6826=DIRECTION ( 'NONE',  ( -0.000000000000000000, -1.000000000000000000, -0.000000000000000000 ) ) ;
#6840=FACE_OUTER_BOUND ( 'NONE', #23619, .T. ) ;
#6870=FACE_OUTER_BOUND ( 'NONE', #7313, .T. ) ;
#6911=EDGE_CURVE ( 'NONE', #48283, #4125, #47087, .T. ) ;
#6912=ORIENTED_EDGE ( 'NONE', *, *, #3335, .F. ) ;
#6922=CARTESIAN_POINT ( 'NONE',  ( -33.52409385541305653, -6.359206544744109735, 52.29999999999998295 ) ) ;
#6926=DIRECTION ( 'NONE',  ( 0.000000000000000000, 0.000000000000000000, 1.000000000000000000 ) ) ;
#6937=VERTEX_POINT ( 'NONE', #21295 ) ;
#6962=EDGE_CURVE ( 'NONE', #43029, #34970, #3293, .T. ) ;
#6985=EDGE_LOOP ( 'NONE', ( #45054, #13090, #35602, #32160, #6912, #30278, #27834, #297 ) ) ;
#7014=ORIENTED_EDGE ( 'NONE', *, *, #30757, .F. ) ;
#7086=CIRCLE ( 'NONE', #5513, 1.050000000000002265 ) ;
#7094=CARTESIAN_POINT ( 'NONE',  ( -7.424093855413048892, -25.10920654474410441, 63.99999999999998579 ) ) ;
#7095=ORIENTED_EDGE ( 'NONE', *, *, #20587, .F. ) ;
#7127=AXIS2_PLACEMENT_3D ( 'NONE', #42213, #11433, #45431 ) ;
#7128=LINE ( 'NONE', #32720, #5528 ) ;
#7132=CARTESIAN_POINT ( 'NONE',  ( -33.52409385541305653, -25.10920654474410441, 52.29999999999998295 ) ) ;
#7168=ADVANCED_FACE ( 'NONE', ( #36226 ), #2020, .F. ) ;
#7198=ORIENTED_EDGE ( 'NONE', *, *, #21519, .F. ) ;
#7199=DIRECTION ( 'NONE',  ( -2.168404344971008375E-16, 0.000000000000000000, 1.000000000000000000 ) ) ;
#7219=DIRECTION ( 'NONE',  ( 0.000000000000000000, 0.000000000000000000, -1.000000000000000000 ) ) ;
#7253=LINE ( 'NONE', #22497, #34471 ) ;
#7277=FACE_OUTER_BOUND ( 'NONE', #33472, .T. ) ;
#7313=EDGE_LOOP ( 'NONE', ( #2415, #6034, #31456, #18092 ) ) ;
#7323=CARTESIAN_POINT ( 'NONE',  ( -28.42409385541305511, -25.10920654474410441, 45.99999999999998579 ) ) ;
#7324=EDGE_CURVE ( 'NONE', #2752, #31166, #8611, .T. ) ;
#7345=DIRECTION ( 'NONE',  ( 0.000000000000000000, 1.000000000000000000, -0.000000000000000000 ) ) ;
#7384=VERTEX_POINT ( 'NONE', #9067 ) ;
#7411=ORIENTED_EDGE ( 'NONE', *, *, #42946, .T. ) ;
#7439=ORIENTED_EDGE ( 'NONE', *, *, #31904, .T. ) ;
#7452=ADVANCED_FACE ( 'NONE', ( #39333, #31706 ), #18985, .T. ) ;
#7491=AXIS2_PLACEMENT_3D ( 'NONE', #19886, #34888, #16161 ) ;
#7524=DIRECTION ( 'NONE',  ( -0.000000000000000000, -1.000000000000000000, -0.000000000000000000 ) ) ;
#7528=EDGE_LOOP ( 'NONE', ( #45871, #33952, #9370, #18364 ) ) ;
#7544=EDGE_LOOP ( 'NONE', ( #3803, #12389, #16459, #30673 ) ) ;
#7551=ORIENTED_EDGE ( 'NONE', *, *, #500, .T. ) ;
#7562=ORIENTED_EDGE ( 'NONE', *, *, #42975, .F. ) ;
#7585=DIRECTION ( 'NONE',  ( 0.000000000000000000, 0.000000000000000000, 1.000000000000000000 ) ) ;
#7592=ORIENTED_EDGE ( 'NONE', *, *, #4205, .T. ) ;
#7641=EDGE_CURVE ( 'NONE', #8993, #10239, #29223, .T. ) ;
#7644=EDGE_CURVE ( 'NONE', #28963, #25288, #29705, .T. ) ;
#7661=VERTEX_POINT ( 'NONE', #26753 ) ;
#7681=LINE ( 'NONE', #41641, #41629 ) ;
#7702=PRESENTATION_STYLE_ASSIGNMENT (( #45855 ) ) ;
#7705=DIRECTION ( 'NONE',  ( 0.000000000000000000, 0.000000000000000000, 1.000000000000000000 ) ) ;
#7721=CARTESIAN_POINT ( 'NONE',  ( -16.94712425470457973, -14.65920654474411045, 52.21286476528345588 ) ) ;
#7740=ORIENTED_EDGE ( 'NONE', *, *, #23504, .T. ) ;
#7791=VECTOR ( 'NONE', #1287, 1000.000000000000000 ) ;
#7812=ORIENTED_EDGE ( 'NONE', *, *, #47313, .T. ) ;
#7830=CARTESIAN_POINT ( 'NONE',  ( -46.92409385541305511, -17.80920654474410370, 62.75000000000000000 ) ) ;
#7867=FACE_OUTER_BOUND ( 'NONE', #15494, .T. ) ;
#7899=ORIENTED_EDGE ( 'NONE', *, *, #41754, .F. ) ;
#7900=ADVANCED_FACE ( 'NONE', ( #42254 ), #11978, .F. ) ;
#7930=CARTESIAN_POINT ( 'NONE',  ( -7.424093855413048892, -27.10920654474410796, 56.99999999999997868 ) ) ;
#7977=CARTESIAN_POINT ( 'NONE',  ( -8.424093855413067544, -8.109206544744111511, 50.49999999999999289 ) ) ;
#7984=CIRCLE ( 'NONE', #41002, 0.3999999999999975797 ) ;
#7987=ORIENTED_EDGE ( 'NONE', *, *, #43381, .F. ) ;
#7998=FACE_OUTER_BOUND ( 'NONE', #42012, .T. ) ;
#8028=EDGE_CURVE ( 'NONE', #6937, #27994, #29165, .T. ) ;
#8047=ORIENTED_EDGE ( 'NONE', *, *, #19993, .F. ) ;
#8048=CARTESIAN_POINT ( 'NONE',  ( -4.424093855413056886, -8.109206544744111511, 50.49999999999999289 ) ) ;
#8050=CARTESIAN_POINT ( 'NONE',  ( -27.42409385541305511, -10.10920654474410618, 63.99999999999998579 ) ) ;
#8090=CARTESIAN_POINT ( 'NONE',  ( -4.924093855413050669, -6.359206544744109735, 47.99999999999998579 ) ) ;
#8117=FACE_OUTER_BOUND ( 'NONE', #19854, .T. ) ;
#8170=ORIENTED_EDGE ( 'NONE', *, *, #29630, .T. ) ;
#8178=DIRECTION ( 'NONE',  ( 0.000000000000000000, 0.000000000000000000, 1.000000000000000000 ) ) ;
#8183=VERTEX_POINT ( 'NONE', #26936 ) ;
#8191=VERTEX_POINT ( 'NONE', #1549 ) ;
#8230=FACE_OUTER_BOUND ( 'NONE', #37923, .T. ) ;
#8235=CARTESIAN_POINT ( 'NONE',  ( -7.924093855413059551, -6.359206544744109735, 47.99999999999998579 ) ) ;
#8251=ADVANCED_FACE ( 'NONE', ( #41954, #20270, #27896 ), #12154, .T. ) ;
#8253=CARTESIAN_POINT ( 'NONE',  ( -26.42409385541305511, -8.109206544744111511, 50.50000000000000000 ) ) ;
#8267=ADVANCED_FACE ( 'NONE', ( #8230 ), #23245, .T. ) ;
#8269=EDGE_CURVE ( 'NONE', #17144, #10239, #25928, .T. ) ;
#8318=DIRECTION ( 'NONE',  ( -1.000000000000000000, 0.000000000000000000, 0.000000000000000000 ) ) ;
#8320=CIRCLE ( 'NONE', #46064, 0.3999999999999975797 ) ;
#8330=CYLINDRICAL_SURFACE ( 'NONE', #5536, 2.000000000000001776 ) ;
#8395=DIRECTION ( 'NONE',  ( 0.000000000000000000, -0.000000000000000000, -1.000000000000000000 ) ) ;
#8421=AXIS2_PLACEMENT_3D ( 'NONE', #29623, #6004, #21027 ) ;
#8423=ORIENTED_EDGE ( 'NONE', *, *, #24903, .F. ) ;
#8424=DIRECTION ( 'NONE',  ( 0.000000000000000000, 1.000000000000000000, 0.000000000000000000 ) ) ;
#8442=EDGE_CURVE ( 'NONE', #42114, #20623, #44617, .T. ) ;
#8451=LINE ( 'NONE', #31340, #5360 ) ;
#8462=AXIS2_PLACEMENT_3D ( 'NONE', #4270, #38219, #22998 ) ;
#8477=CARTESIAN_POINT ( 'NONE',  ( -45.92409385541305511, -17.80920654474410370, 70.50000000000000000 ) ) ;
#8497=ORIENTED_EDGE ( 'NONE', *, *, #7644, .F. ) ;
#8510=SHAPE_DEFINITION_REPRESENTATION ( #35058, #46513 ) ;
#8519=ORIENTED_EDGE ( 'NONE', *, *, #39944, .T. ) ;
#8525=CIRCLE ( 'NONE', #9298, 1.999999999999994893 ) ;
#8526=VECTOR ( 'NONE', #46495, 1000.000000000000000 ) ;
#8532=DIRECTION ( 'NONE',  ( 0.000000000000000000, 1.000000000000000000, -0.000000000000000000 ) ) ;
#8579=ADVANCED_FACE ( 'NONE', ( #13525 ), #24645, .T. ) ;
#8605=ORIENTED_EDGE ( 'NONE', *, *, #10303, .F. ) ;
#8611=CIRCLE ( 'NONE', #21151, 1.500000000000008216 ) ;
#8647=FACE_OUTER_BOUND ( 'NONE', #31555, .T. ) ;
#8661=CARTESIAN_POINT ( 'NONE',  ( -26.42409385541305511, -15.80920654474410725, 47.99999999999997868 ) ) ;
#8674=EDGE_CURVE ( 'NONE', #2631, #28641, #13042, .T. ) ;
#8696=DIRECTION ( 'NONE',  ( 2.775557561562888984E-15, 0.000000000000000000, -1.000000000000000000 ) ) ;
#8702=VECTOR ( 'NONE', #25346, 1000.000000000000000 ) ;
#8705=CARTESIAN_POINT ( 'NONE',  ( -50.42409385541304800, -15.80920654474410725, 56.99999999999999289 ) ) ;
#8714=CYLINDRICAL_SURFACE ( 'NONE', #22630, 0.5000000000000004441 ) ;
#8723=ORIENTED_EDGE ( 'NONE', *, *, #45646, .F. ) ;
#8746=PRODUCT ( 'Base Cast Iron Chassis Plate', 'Base Cast Iron Chassis Plate', '', ( #38049 ) ) ;
#8782=AXIS2_PLACEMENT_3D ( 'NONE', #2959, #26118, #44354 ) ;
#8787=ORIENTED_EDGE ( 'NONE', *, *, #23943, .T. ) ;
#8808=AXIS2_PLACEMENT_3D ( 'NONE', #27187, #30894, #16322 ) ;
#8821=CARTESIAN_POINT ( 'NONE',  ( -13.92409385541305511, -10.60920654474410618, 81.99999999999998579 ) ) ;
#8860=ADVANCED_FACE ( 'NONE', ( #959, #8117 ), #30526, .F. ) ;
#8888=DIRECTION ( 'NONE',  ( 1.000000000000000000, 0.000000000000000000, 8.260587980841940012E-17 ) ) ;
#8892=DIRECTION ( 'NONE',  ( 0.000000000000000000, 0.000000000000000000, 1.000000000000000000 ) ) ;
#8900=CARTESIAN_POINT ( 'NONE',  ( -50.42409385541304800, -25.10920654474410441, 63.99999999999998579 ) ) ;
#8904=PLANE ( 'NONE',  #19204 ) ;
#8945=ORIENTED_EDGE ( 'NONE', *, *, #6911, .T. ) ;
#8950=ADVANCED_FACE ( 'NONE', ( #5140 ), #9805, .T. ) ;
#8957=ORIENTED_EDGE ( 'NONE', *, *, #29794, .T. ) ;
#8958=DIRECTION ( 'NONE',  ( -0.000000000000000000, 0.000000000000000000, 1.000000000000000000 ) ) ;
#8972=CARTESIAN_POINT ( 'NONE',  ( -9.424093855413055110, -25.10920654474410441, 54.99999999999997868 ) ) ;
#8974=ORIENTED_EDGE ( 'NONE', *, *, #2600, .T. ) ;
#8986=ORIENTED_EDGE ( 'NONE', *, *, #11769, .F. ) ;
#8993=VERTEX_POINT ( 'NONE', #124 ) ;
#9010=DIRECTION ( 'NONE',  ( 1.000000000000000000, -0.000000000000000000, -0.000000000000000000 ) ) ;
#9013=ADVANCED_FACE ( 'NONE', ( #15346 ), #41467, .T. ) ;
#9021=EDGE_LOOP ( 'NONE', ( #151, #22973, #34146, #22347 ) ) ;
#9059=AXIS2_PLACEMENT_3D ( 'NONE', #26644, #26390, #41405 ) ;
#9060=CARTESIAN_POINT ( 'NONE',  ( -33.52409385541305653, -8.109206544744111511, 51.54999999999998295 ) ) ;
#9064=AXIS2_PLACEMENT_3D ( 'NONE', #28241, #6315, #17124 ) ;
#9067=CARTESIAN_POINT ( 'NONE',  ( -48.42409385541304800, -25.10920654474410441, 81.99999999999998579 ) ) ;
#9126=LINE ( 'NONE', #19962, #10948 ) ;
#9130=CARTESIAN_POINT ( 'NONE',  ( -48.42409385541304800, -27.10920654474410796, 81.99999999999998579 ) ) ;
#9150=VERTEX_POINT ( 'NONE', #28640 ) ;
#9160=DIRECTION ( 'NONE',  ( 0.000000000000000000, 1.000000000000000000, -0.000000000000000000 ) ) ;
#9244=DIRECTION ( 'NONE',  ( 0.000000000000000000, 0.000000000000000000, 1.000000000000000000 ) ) ;
#9252=LINE ( 'NONE', #19855, #31327 ) ;
#9264=VECTOR ( 'NONE', #3378, 1000.000000000000000 ) ;
#9275=VECTOR ( 'NONE', #16306, 1000.000000000000000 ) ;
#9293=AXIS2_PLACEMENT_3D ( 'NONE', #15776, #30348, #30832 ) ;
#9297=CARTESIAN_POINT ( 'NONE',  ( -26.92409385541305511, -6.359206544744109735, 47.99999999999997868 ) ) ;
#9298=AXIS2_PLACEMENT_3D ( 'NONE', #1541, #42682, #19786 ) ;
#9321=DIRECTION ( 'NONE',  ( 1.000000000000000000, 0.000000000000000000, 0.000000000000000000 ) ) ;
#9323=DIRECTION ( 'NONE',  ( 0.000000000000000000, 0.000000000000000000, 1.000000000000000000 ) ) ;
#9338=AXIS2_PLACEMENT_3D ( 'NONE', #18065, #9974, #17096 ) ;
#9348=ORIENTED_EDGE ( 'NONE', *, *, #13591, .T. ) ;
#9370=ORIENTED_EDGE ( 'NONE', *, *, #14520, .T. ) ;
#9420=VERTEX_POINT ( 'NONE', #43334 ) ;
#9438=AXIS2_PLACEMENT_3D ( 'NONE', #46417, #31873, #5783 ) ;
#9447=EDGE_LOOP ( 'NONE', ( #45798, #47356, #11485, #14983 ) ) ;
#9495=EDGE_CURVE ( 'NONE', #44063, #38493, #32705, .T. ) ;
#9524=AXIS2_PLACEMENT_3D ( 'NONE', #47657, #48140, #17835 ) ;
#9569=ORIENTED_EDGE ( 'NONE', *, *, #42763, .F. ) ;
#9575=ADVANCED_FACE ( 'NONE', ( #4379 ), #33413, .F. ) ;
#9583=CIRCLE ( 'NONE', #30803, 2.500000000000002220 ) ;
#9629=CARTESIAN_POINT ( 'NONE',  ( -45.92409385541305511, -17.80920654474410370, 70.50000000000000000 ) ) ;
#9680=LINE ( 'NONE', #5967, #46489 ) ;
#9713=ADVANCED_FACE ( 'NONE', ( #45992 ), #12492, .F. ) ;
#9723=FACE_OUTER_BOUND ( 'NONE', #35253, .T. ) ;
#9737=VECTOR ( 'NONE', #48040, 1000.000000000000000 ) ;
#9746=LINE ( 'NONE', #13159, #23933 ) ;
#9751=EDGE_CURVE ( 'NONE', #1645, #17537, #12249, .T. ) ;
#9781=DIRECTION ( 'NONE',  ( 0.000000000000000000, 1.000000000000000000, -0.000000000000000000 ) ) ;
#9783=ORIENTED_EDGE ( 'NONE', *, *, #2394, .T. ) ;
#9788=ORIENTED_EDGE ( 'NONE', *, *, #15735, .F. ) ;
#9799=CARTESIAN_POINT ( 'NONE',  ( -17.42409385541305511, -14.80920654474410725, 48.99999999999997868 ) ) ;
#9805=PLANE ( 'NONE',  #18064 ) ;
#9816=CARTESIAN_POINT ( 'NONE',  ( -28.42409385541305511, -6.859206544744110623, 52.99999999999997158 ) ) ;
#9832=FACE_OUTER_BOUND ( 'NONE', #36532, .T. ) ;
#9842=ORIENTED_EDGE ( 'NONE', *, *, #21563, .F. ) ;
#9856=ORIENTED_EDGE ( 'NONE', *, *, #3273, .T. ) ;
#9877=DIRECTION ( 'NONE',  ( -0.000000000000000000, -0.000000000000000000, 1.000000000000000000 ) ) ;
#9900=CARTESIAN_POINT ( 'NONE',  ( -46.92409385541305511, -17.80920654474410370, 60.24999999999999289 ) ) ;
#9924=LINE ( 'NONE', #24941, #10559 ) ;
#9943=CARTESIAN_POINT ( 'NONE',  ( -42.07024770156689897, -25.10920654474410441, 65.83076923076922071 ) ) ;
#9947=CARTESIAN_POINT ( 'NONE',  ( -9.424093855413051557, -25.10920654474410441, 77.00000000000000000 ) ) ;
#9948=EDGE_CURVE ( 'NONE', #11779, #744, #45492, .T. ) ;
#9962=VERTEX_POINT ( 'NONE', #39296 ) ;
#9974=DIRECTION ( 'NONE',  ( 1.927470528863119542E-16, 0.000000000000000000, -1.000000000000000000 ) ) ;
#9997=DIRECTION ( 'NONE',  ( 0.000000000000000000, 1.000000000000000000, 0.000000000000000000 ) ) ;
#10002=EDGE_CURVE ( 'NONE', #30760, #37795, #39351, .T. ) ;
#10004=DIRECTION ( 'NONE',  ( 0.000000000000000000, 1.000000000000000000, -0.000000000000000000 ) ) ;
#10015=ORIENTED_EDGE ( 'NONE', *, *, #21286, .F. ) ;
#10024=FACE_OUTER_BOUND ( 'NONE', #34646, .T. ) ;
#10025=UNCERTAINTY_MEASURE_WITH_UNIT (LENGTH_MEASURE( 1.000000000000000082E-05 ), #43856, 'distance_accuracy_value', 'NONE');
#10033=TOROIDAL_SURFACE ( 'NONE', #18655, 1.499999999999998224, 0.5000000000000000000 ) ;
#10047=VECTOR ( 'NONE', #29408, 1000.000000000000000 ) ;
#10064=ORIENTED_EDGE ( 'NONE', *, *, #13548, .F. ) ;
#10070=CIRCLE ( 'NONE', #47821, 0.5000000000000004441 ) ;
#10077=LINE ( 'NONE', #36398, #20929 ) ;
#10087=ADVANCED_FACE ( 'NONE', ( #7277 ), #2597, .F. ) ;
#10093=ORIENTED_EDGE ( 'NONE', *, *, #44150, .F. ) ;
#10123=CARTESIAN_POINT ( 'NONE',  ( -4.424093855413056886, -8.109206544744111511, 50.49999999999999289 ) ) ;
#10130=CARTESIAN_POINT ( 'NONE',  ( -8.424093855413063991, -15.80920654474410725, 48.99999999999997868 ) ) ;
#10151=CARTESIAN_POINT ( 'NONE',  ( -26.42409385541305511, -6.359206544744109735, 52.99999999999997158 ) ) ;
#10165=LINE ( 'NONE', #17766, #14192 ) ;
#10175=EDGE_CURVE ( 'NONE', #733, #1179, #3959, .T. ) ;
#10197=PLANE ( 'NONE',  #34660 ) ;
#10204=DIRECTION ( 'NONE',  ( -1.000000000000000000, 0.000000000000000000, 0.000000000000000000 ) ) ;
#10213=ORIENTED_EDGE ( 'NONE', *, *, #1284, .T. ) ;
#10226=DIRECTION ( 'NONE',  ( -1.000000000000000000, 0.000000000000000000, -0.000000000000000000 ) ) ;
#10228=VERTEX_POINT ( 'NONE', #30662 ) ;
#10239=VERTEX_POINT ( 'NONE', #601 ) ;
#10285=DIRECTION ( 'NONE',  ( 0.000000000000000000, 0.000000000000000000, 1.000000000000000000 ) ) ;
#10303=EDGE_CURVE ( 'NONE', #9962, #20146, #17330, .T. ) ;
#10313=ADVANCED_FACE ( 'NONE', ( #20289 ), #5034, .T. ) ;
#10316=EDGE_CURVE ( 'NONE', #23071, #18406, #39488, .T. ) ;
#10317=DIRECTION ( 'NONE',  ( 1.000000000000000000, 0.000000000000000000, -8.260587980841940012E-17 ) ) ;
#10323=CARTESIAN_POINT ( 'NONE',  ( -14.92409385541305333, -14.80920654474410725, 81.99999999999998579 ) ) ;
#10348=ORIENTED_EDGE ( 'NONE', *, *, #18691, .T. ) ;
#10354=VECTOR ( 'NONE', #6011, 1000.000000000000000 ) ;
#10360=VECTOR ( 'NONE', #21630, 1000.000000000000000 ) ;
#10379=CIRCLE ( 'NONE', #31615, 2.000000000000001776 ) ;
#10384=FACE_OUTER_BOUND ( 'NONE', #44448, .T. ) ;
#10414=FACE_OUTER_BOUND ( 'NONE', #39840, .T. ) ;
#10421=CARTESIAN_POINT ( 'NONE',  ( -27.42409385541305511, -25.10920654474410441, 63.99999999999998579 ) ) ;
#10431=VERTEX_POINT ( 'NONE', #21979 ) ;
#10475=AXIS2_PLACEMENT_3D ( 'NONE', #35786, #17063, #13372 ) ;
#10490=CARTESIAN_POINT ( 'NONE',  ( -4.424093855413056886, -25.10920654474410441, 79.99999999999998579 ) ) ;
#10496=CARTESIAN_POINT ( 'NONE',  ( -41.15852941833841783, -25.10920654474410441, 54.99999999999997868 ) ) ;
#10527=DIRECTION ( 'NONE',  ( 0.000000000000000000, 0.000000000000000000, 1.000000000000000000 ) ) ;
#10539=CARTESIAN_POINT ( 'NONE',  ( -45.92409385541305511, -17.80920654474410370, 70.50000000000000000 ) ) ;
#10552=ADVANCED_FACE ( 'NONE', ( #44639 ), #44896, .F. ) ;
#10556=EDGE_LOOP ( 'NONE', ( #28980, #9569, #47736, #40219 ) ) ;
#10559=VECTOR ( 'NONE', #39959, 1000.000000000000000 ) ;
#10560=DIRECTION ( 'NONE',  ( -0.000000000000000000, -1.000000000000000000, -0.000000000000000000 ) ) ;
#10572=ORIENTED_EDGE ( 'NONE', *, *, #46589, .T. ) ;
#10574=EDGE_CURVE ( 'NONE', #20146, #9962, #1633, .T. ) ;
#10587=VERTEX_POINT ( 'NONE', #17173 ) ;
#10596=AXIS2_PLACEMENT_3D ( 'NONE', #40913, #25419, #22452 ) ;
#10621=ADVANCED_FACE ( 'NONE', ( #47241 ), #43055, .F. ) ;
#10692=DIRECTION ( 'NONE',  ( -0.000000000000000000, -0.000000000000000000, 1.000000000000000000 ) ) ;
#10697=AXIS2_PLACEMENT_3D ( 'NONE', #34265, #8424, #12355 ) ;
#10707=ORIENTED_EDGE ( 'NONE', *, *, #17494, .F. ) ;
#10726=DIRECTION ( 'NONE',  ( 0.000000000000000000, 0.000000000000000000, 1.000000000000000000 ) ) ;
#10733=ORIENTED_EDGE ( 'NONE', *, *, #6613, .F. ) ;
#10764=AXIS2_PLACEMENT_3D ( 'NONE', #24367, #13499, #40753 ) ;
#10769=EDGE_CURVE ( 'NONE', #26221, #36791, #20524, .T. ) ;
#10774=CARTESIAN_POINT ( 'NONE',  ( -30.42409385541305156, -6.859206544744110623, 47.99999999999997868 ) ) ;
#10792=VECTOR ( 'NONE', #31789, 1000.000000000000000 ) ;
#10825=CARTESIAN_POINT ( 'NONE',  ( -13.92409385541305511, -10.10920654474410618, 81.49999999999998579 ) ) ;
#10834=CARTESIAN_POINT ( 'NONE',  ( -27.42409385541305156, -25.10920654474410441, 74.99999999999998579 ) ) ;
#10844=DIRECTION ( 'NONE',  ( 0.000000000000000000, 1.000000000000000000, -0.000000000000000000 ) ) ;
#10879=AXIS2_PLACEMENT_3D ( 'NONE', #11358, #45345, #4223 ) ;
#10901=ADVANCED_FACE ( 'NONE', ( #27013 ), #4362, .F. ) ;
#10927=FACE_OUTER_BOUND ( 'NONE', #39345, .T. ) ;
#10948=VECTOR ( 'NONE', #24638, 1000.000000000000000 ) ;
#10969=LINE ( 'NONE', #36797, #11572 ) ;
#11008=LINE ( 'NONE', #26032, #20306 ) ;
#11025=PLANE ( 'NONE',  #48037 ) ;
#11033=ORIENTED_EDGE ( 'NONE', *, *, #15705, .F. ) ;
#11065=CIRCLE ( 'NONE', #32297, 1.250000000000001110 ) ;
#11089=ADVANCED_FACE ( 'NONE', ( #14860 ), #24467, .T. ) ;
#11101=ORIENTED_EDGE ( 'NONE', *, *, #46174, .F. ) ;
#11113=DIRECTION ( 'NONE',  ( 0.000000000000000000, 0.000000000000000000, 1.000000000000000000 ) ) ;
#11142=CARTESIAN_POINT ( 'NONE',  ( -35.32409385541306079, -25.10920654474410441, 48.79999999999998295 ) ) ;
#11146=CARTESIAN_POINT ( 'NONE',  ( -33.95962776134579286, -8.109206544744111511, 50.50000000000000000 ) ) ;
#11156=ADVANCED_FACE ( 'NONE', ( #2830 ), #21328, .T. ) ;
#11187=VECTOR ( 'NONE', #23700, 1000.000000000000000 ) ;
#11237=EDGE_CURVE ( 'NONE', #27788, #30260, #18833, .T. ) ;
#11264=VERTEX_POINT ( 'NONE', #19564 ) ;
#11302=CARTESIAN_POINT ( 'NONE',  ( -38.65852941833841783, -25.10920654474410441, 78.99999999999998579 ) ) ;
#11319=FACE_OUTER_BOUND ( 'NONE', #9021, .T. ) ;
#11358=CARTESIAN_POINT ( 'NONE',  ( -17.42409385541305511, -14.80920654474410725, 47.99999999999998579 ) ) ;
#11379=CARTESIAN_POINT ( 'NONE',  ( -9.424093855413055110, -27.10920654474410796, 56.99999999999997868 ) ) ;
#11393=VERTEX_POINT ( 'NONE', #40689 ) ;
#11398=DIRECTION ( 'NONE',  ( 0.000000000000000000, 0.000000000000000000, 1.000000000000000000 ) ) ;
#11405=PLANE ( 'NONE',  #8462 ) ;
#11410=DIRECTION ( 'NONE',  ( 2.181982678098338148E-16, 0.000000000000000000, -1.000000000000000000 ) ) ;
#11433=DIRECTION ( 'NONE',  ( -1.000000000000000000, 0.000000000000000000, 0.000000000000000000 ) ) ;
#11453=DIRECTION ( 'NONE',  ( 0.000000000000000000, 1.000000000000000000, -0.000000000000000000 ) ) ;
#11480=VERTEX_POINT ( 'NONE', #4484 ) ;
#11485=ORIENTED_EDGE ( 'NONE', *, *, #15293, .F. ) ;
#11495=CARTESIAN_POINT ( 'NONE',  ( -16.92409385541305511, -14.80920654474410547, 48.99999999999997868 ) ) ;
#11549=DIRECTION ( 'NONE',  ( -1.000000000000000000, 0.000000000000000000, 0.000000000000000000 ) ) ;
#11572=VECTOR ( 'NONE', #32238, 1000.000000000000000 ) ;
#11584=CARTESIAN_POINT ( 'NONE',  ( -27.42409385541305511, -15.80920654474410725, 48.99999999999997868 ) ) ;
#11603=ORIENTED_EDGE ( 'NONE', *, *, #21811, .T. ) ;
#11606=ORIENTED_EDGE ( 'NONE', *, *, #48142, .F. ) ;
#11624=VECTOR ( 'NONE', #20027, 1000.000000000000000 ) ;
#11669=DIRECTION ( 'NONE',  ( 1.000000000000000000, 0.000000000000000000, 1.927470528863119295E-16 ) ) ;
#11680=DIRECTION ( 'NONE',  ( 0.000000000000000000, 0.000000000000000000, 1.000000000000000000 ) ) ;
#11698=DIRECTION ( 'NONE',  ( 0.000000000000000000, 1.000000000000000000, 0.000000000000000000 ) ) ;
#11732=VERTEX_POINT ( 'NONE', #39668 ) ;
#11743=CARTESIAN_POINT ( 'NONE',  ( -28.42409385541305511, -6.359206544744109735, 47.99999999999997868 ) ) ;
#11768=AXIS2_PLACEMENT_3D ( 'NONE', #2276, #20752, #5970 ) ;
#11769=EDGE_CURVE ( 'NONE', #33284, #36353, #7984, .T. ) ;
#11774=CARTESIAN_POINT ( 'NONE',  ( -17.79490377976783932, -14.65920654474411045, 47.99999999999998579 ) ) ;
#11779=VERTEX_POINT ( 'NONE', #13780 ) ;
#11784=ORIENTED_EDGE ( 'NONE', *, *, #3328, .T. ) ;
#11832=DIRECTION ( 'NONE',  ( 0.000000000000000000, 0.000000000000000000, 1.000000000000000000 ) ) ;
#11842=CLOSED_SHELL ( 'NONE', ( #14405, #27267, #11947, #1056, #10901, #47344, #43346, #26441, #5877, #10313, #29245, #28891, #24227, #7452, #26996, #48492, #8860, #39497, #1467, #41355, #31308, #8267, #17385, #36199, #41468, #44530, #40702, #10621, #42822, #9575, #1377, #43250, #9713, #45573, #28078, #8950, #3781, #27630, #18459, #14956, #18440, #46651, #33775, #3536, #2112, #17095, #10552, #38064, #38343, #8251, #24487, #11156, #25373, #21876, #37241, #16412, #948, #30034, #6349, #10087, #41112, #8579, #41596, #41675, #7168, #1350, #20948, #62, #21700, #7900, #5053, #16438, #34418, #11089, #2334, #6329, #667, #22105, #27508, #31787, #17796, #35593, #47613, #9013, #34960 ) ) ;
#11886=AXIS2_PLACEMENT_3D ( 'NONE', #18899, #13956, #44053 ) ;
#11898=ORIENTED_EDGE ( 'NONE', *, *, #9751, .T. ) ;
#11909=DIRECTION ( 'NONE',  ( 0.000000000000000000, 0.000000000000000000, -1.000000000000000000 ) ) ;
#11915=CARTESIAN_POINT ( 'NONE',  ( -8.424093855413063991, -8.109206544744111511, 49.24999999999999289 ) ) ;
#11933=VECTOR ( 'NONE', #11669, 1000.000000000000000 ) ;
#11934=DIRECTION ( 'NONE',  ( 1.000000000000000000, 0.000000000000000000, 0.000000000000000000 ) ) ;
#11947=ADVANCED_FACE ( 'NONE', ( #24114 ), #20426, .F. ) ;
#11968=CARTESIAN_POINT ( 'NONE',  ( -7.924093855413059551, -6.859206544744110623, 47.99999999999998579 ) ) ;
#11978=CYLINDRICAL_SURFACE ( 'NONE', #31375, 1.050000000000002265 ) ;
#11984=ORIENTED_EDGE ( 'NONE', *, *, #25558, .F. ) ;
#12012=DIRECTION ( 'NONE',  ( 0.000000000000000000, 0.000000000000000000, -1.000000000000000000 ) ) ;
#12018=CARTESIAN_POINT ( 'NONE',  ( -38.65852941833841783, -25.10920654474410441, 76.99999999999998579 ) ) ;
#12046=DIRECTION ( 'NONE',  ( 0.000000000000000000, 0.000000000000000000, -1.000000000000000000 ) ) ;
#12091=DIRECTION ( 'NONE',  ( -0.000000000000000000, -1.000000000000000000, -0.000000000000000000 ) ) ;
#12097=VERTEX_POINT ( 'NONE', #47724 ) ;
#12113=ORIENTED_EDGE ( 'NONE', *, *, #25640, .T. ) ;
#12122=EDGE_CURVE ( 'NONE', #48317, #30462, #40338, .T. ) ;
#12137=ORIENTED_EDGE ( 'NONE', *, *, #23873, .F. ) ;
#12154=PLANE ( 'NONE',  #44007 ) ;
#12188=CARTESIAN_POINT ( 'NONE',  ( -50.42509385541305988, -8.109206544744111511, 49.44999999999998863 ) ) ;
#12226=LINE ( 'NONE', #35355, #12941 ) ;
#12249=LINE ( 'NONE', #31448, #26779 ) ;
#12261=ORIENTED_EDGE ( 'NONE', *, *, #1728, .T. ) ;
#12279=CARTESIAN_POINT ( 'NONE',  ( -27.42409385541305511, -25.10920654474410441, 56.99999999999999289 ) ) ;
#12295=DIRECTION ( 'NONE',  ( -0.000000000000000000, 1.000000000000000000, -0.000000000000000000 ) ) ;
#12318=VECTOR ( 'NONE', #3084, 1000.000000000000000 ) ;
#12355=DIRECTION ( 'NONE',  ( 0.000000000000000000, -0.000000000000000000, 1.000000000000000000 ) ) ;
#12368=ORIENTED_EDGE ( 'NONE', *, *, #3335, .T. ) ;
#12389=ORIENTED_EDGE ( 'NONE', *, *, #43570, .T. ) ;
#12478=DIRECTION ( 'NONE',  ( 0.000000000000000000, 0.000000000000000000, -1.000000000000000000 ) ) ;
#12486=LINE ( 'NONE', #1157, #36150 ) ;
#12491=DIRECTION ( 'NONE',  ( 0.000000000000000000, 0.000000000000000000, 1.000000000000000000 ) ) ;
#12492=CYLINDRICAL_SURFACE ( 'NONE', #21293, 2.000000000000001776 ) ;
#12520=LINE ( 'NONE', #5388, #23613 ) ;
#12522=AXIS2_PLACEMENT_3D ( 'NONE', #17215, #12804, #43092 ) ;
#12535=DIRECTION ( 'NONE',  ( 0.000000000000000000, 0.000000000000000000, -1.000000000000000000 ) ) ;
#12592=ORIENTED_EDGE ( 'NONE', *, *, #19217, .T. ) ;
#12593=EDGE_LOOP ( 'NONE', ( #42237, #20653, #40778, #24091 ) ) ;
#12604=ORIENTED_EDGE ( 'NONE', *, *, #30706, .F. ) ;
#12610=CARTESIAN_POINT ( 'NONE',  ( -4.924093855413054222, -6.359206544744109735, 63.99999999999998579 ) ) ;
#12638=ADVANCED_BREP_SHAPE_REPRESENTATION ( '', ( #48569, #29031 ), #39238 ) ;
#12687=TOROIDAL_SURFACE ( 'NONE', #40222, 1.499999999999998224, 0.5000000000000000000 ) ;
#12688=LINE ( 'NONE', #38541, #30575 ) ;
#12717=CARTESIAN_POINT ( 'NONE',  ( -43.17409385541305511, -15.80920654474410725, 56.99999999999999289 ) ) ;
#12722=VERTEX_POINT ( 'NONE', #14021 ) ;
#12728=ORIENTED_EDGE ( 'NONE', *, *, #26187, .F. ) ;
#12735=EDGE_CURVE ( 'NONE', #10228, #5216, #17810, .T. ) ;
#12757=FACE_OUTER_BOUND ( 'NONE', #10556, .T. ) ;
#12779=ORIENTED_EDGE ( 'NONE', *, *, #2394, .F. ) ;
#12781=DIRECTION ( 'NONE',  ( 2.181982678098338148E-16, 0.000000000000000000, -1.000000000000000000 ) ) ;
#12804=DIRECTION ( 'NONE',  ( 0.000000000000000000, 1.000000000000000000, -0.000000000000000000 ) ) ;
#12813=DIRECTION ( 'NONE',  ( 0.000000000000000000, -0.000000000000000000, 1.000000000000000000 ) ) ;
#12833=ORIENTED_EDGE ( 'NONE', *, *, #31880, .T. ) ;
#12835=DIRECTION ( 'NONE',  ( -0.000000000000000000, -1.000000000000000000, -0.000000000000000000 ) ) ;
#12855=CARTESIAN_POINT ( 'NONE',  ( -30.42409385541305156, -8.109206544744111511, 51.75000000000000711 ) ) ;
#12860=DIRECTION ( 'NONE',  ( 0.000000000000000000, 1.000000000000000000, -0.000000000000000000 ) ) ;
#12878=CARTESIAN_POINT ( 'NONE',  ( -13.92409385541305511, -10.60920654474410618, 80.49999999999998579 ) ) ;
#12893=CYLINDRICAL_SURFACE ( 'NONE', #6768, 2.000000000000001776 ) ;
#12905=VECTOR ( 'NONE', #42644, 1000.000000000000000 ) ;
#12913=EDGE_CURVE ( 'NONE', #25709, #18406, #4232, .T. ) ;
#12925=DIRECTION ( 'NONE',  ( -1.000000000000000000, 0.000000000000000000, 9.637352644315596475E-17 ) ) ;
#12932=ORIENTED_EDGE ( 'NONE', *, *, #3580, .F. ) ;
#12937=CARTESIAN_POINT ( 'NONE',  ( -48.42409385541304800, -27.10920654474410796, 45.99999999999998579 ) ) ;
#12938=DIRECTION ( 'NONE',  ( 0.000000000000000000, 0.000000000000000000, -1.000000000000000000 ) ) ;
#12941=VECTOR ( 'NONE', #5088, 1000.000000000000000 ) ;
#12986=VERTEX_POINT ( 'NONE', #5693 ) ;
#12991=CARTESIAN_POINT ( 'NONE',  ( -28.42409385541305511, -25.10920654474410441, 52.99999999999997158 ) ) ;
#13017=EDGE_CURVE ( 'NONE', #41929, #26221, #31539, .T. ) ;
#13026=DIRECTION ( 'NONE',  ( -1.000000000000000000, 0.000000000000000000, 0.000000000000000000 ) ) ;
#13042=LINE ( 'NONE', #20700, #27505 ) ;
#13050=CARTESIAN_POINT ( 'NONE',  ( -33.52409385541305653, -6.359206544744109735, 51.54999999999998295 ) ) ;
#13061=CARTESIAN_POINT ( 'NONE',  ( -35.32409385541306079, -8.109206544744111511, 49.44999999999998863 ) ) ;
#13070=EDGE_CURVE ( 'NONE', #33767, #43808, #5919, .T. ) ;
#13076=DIRECTION ( 'NONE',  ( 0.000000000000000000, 0.000000000000000000, -1.000000000000000000 ) ) ;
#13089=CARTESIAN_POINT ( 'NONE',  ( -18.92409385541305511, -15.80920654474410725, 52.21286476528345588 ) ) ;
#13090=ORIENTED_EDGE ( 'NONE', *, *, #2839, .F. ) ;
#13159=CARTESIAN_POINT ( 'NONE',  ( -27.42409385541305511, -25.10920654474410441, 81.99999999999998579 ) ) ;
#13180=DIRECTION ( 'NONE',  ( 1.000000000000000000, 0.000000000000000000, 0.000000000000000000 ) ) ;
#13185=CYLINDRICAL_SURFACE ( 'NONE', #35125, 2.000000000000008882 ) ;
#13207=ORIENTED_EDGE ( 'NONE', *, *, #37086, .F. ) ;
#13225=DIRECTION ( 'NONE',  ( -2.168404344971008375E-16, -0.000000000000000000, 1.000000000000000000 ) ) ;
#13251=CARTESIAN_POINT ( 'NONE',  ( -8.424093855413060439, -6.859206544744110623, 47.99999999999998579 ) ) ;
#13260=ORIENTED_EDGE ( 'NONE', *, *, #21333, .T. ) ;
#13268=DIRECTION ( 'NONE',  ( -0.000000000000000000, -1.000000000000000000, -0.000000000000000000 ) ) ;
#13273=CARTESIAN_POINT ( 'NONE',  ( -17.82409385541305369, -14.80920654474410725, 48.99999999999997868 ) ) ;
#13275=ORIENTED_EDGE ( 'NONE', *, *, #18531, .F. ) ;
#13305=AXIS2_PLACEMENT_3D ( 'NONE', #28635, #46864, #2283 ) ;
#13351=EDGE_CURVE ( 'NONE', #17537, #17620, #16684, .T. ) ;
#13372=DIRECTION ( 'NONE',  ( 1.000000000000000000, 0.000000000000000000, 0.000000000000000000 ) ) ;
#13385=EDGE_LOOP ( 'NONE', ( #6247, #22303, #12779, #25597 ) ) ;
#13487=DIRECTION ( 'NONE',  ( -0.000000000000000000, -1.000000000000000000, -0.000000000000000000 ) ) ;
#13499=DIRECTION ( 'NONE',  ( -1.000000000000000000, -0.000000000000000000, -0.000000000000000000 ) ) ;
#13508=CARTESIAN_POINT ( 'NONE',  ( -20.92409385541305511, -10.10920654474410618, 81.99999999999998579 ) ) ;
#13525=FACE_OUTER_BOUND ( 'NONE', #1363, .T. ) ;
#13526=LINE ( 'NONE', #20204, #32088 ) ;
#13531=LINE ( 'NONE', #28578, #1445 ) ;
#13534=ORIENTED_EDGE ( 'NONE', *, *, #17376, .F. ) ;
#13537=EDGE_CURVE ( 'NONE', #30092, #32365, #18579, .T. ) ;
#13548=EDGE_CURVE ( 'NONE', #24671, #42423, #25308, .T. ) ;
#13561=DIRECTION ( 'NONE',  ( 2.775557561562888984E-15, 0.000000000000000000, -1.000000000000000000 ) ) ;
#13588=DIRECTION ( 'NONE',  ( -1.000000000000000000, 0.000000000000000000, 0.000000000000000000 ) ) ;
#13591=EDGE_CURVE ( 'NONE', #27994, #41987, #37496, .T. ) ;
#13625=DIRECTION ( 'NONE',  ( -1.000000000000000000, 0.000000000000000000, 0.000000000000000000 ) ) ;
#13645=DIRECTION ( 'NONE',  ( 0.000000000000000000, 1.000000000000000000, -0.000000000000000000 ) ) ;
#13676=ORIENTED_EDGE ( 'NONE', *, *, #1937, .T. ) ;
#13703=EDGE_CURVE ( 'NONE', #37795, #42591, #24170, .T. ) ;
#13717=CARTESIAN_POINT ( 'NONE',  ( -35.32409385541306079, -25.10920654474410441, 48.79999999999998295 ) ) ;
#13740=FACE_OUTER_BOUND ( 'NONE', #37412, .T. ) ;
#13746=EDGE_CURVE ( 'NONE', #10431, #32365, #42515, .T. ) ;
#13748=VERTEX_POINT ( 'NONE', #5577 ) ;
#13780=CARTESIAN_POINT ( 'NONE',  ( -17.02409385541305653, -14.80920654474410725, 48.99999999999997868 ) ) ;
#13794=CARTESIAN_POINT ( 'NONE',  ( -27.42409385541305511, -25.10920654474410441, 54.99999999999997868 ) ) ;
#13815=ORIENTED_EDGE ( 'NONE', *, *, #6199, .T. ) ;
#13868=VECTOR ( 'NONE', #31780, 1000.000000000000000 ) ;
#13869=CIRCLE ( 'NONE', #47709, 0.5000000000000004441 ) ;
#13879=PLANE ( 'NONE',  #5400 ) ;
#13884=ORIENTED_EDGE ( 'NONE', *, *, #12913, .F. ) ;
#13886=ORIENTED_EDGE ( 'NONE', *, *, #22218, .F. ) ;
#13898=CARTESIAN_POINT ( 'NONE',  ( -6.424093855413058662, -6.859206544744110623, 52.99999999999998579 ) ) ;
#13922=ORIENTED_EDGE ( 'NONE', *, *, #32918, .T. ) ;
#13947=ORIENTED_EDGE ( 'NONE', *, *, #46888, .T. ) ;
#13956=DIRECTION ( 'NONE',  ( 0.000000000000000000, 0.000000000000000000, 1.000000000000000000 ) ) ;
#13988=CARTESIAN_POINT ( 'NONE',  ( -30.42409385541305156, -6.859206544744110623, 47.99999999999997868 ) ) ;
#14021=CARTESIAN_POINT ( 'NONE',  ( -13.92409385541305511, -25.10920654474410441, 78.99999999999998579 ) ) ;
#14022=EDGE_CURVE ( 'NONE', #19972, #26269, #24163, .T. ) ;
#14117=ORIENTED_EDGE ( 'NONE', *, *, #16754, .F. ) ;
#14146=EDGE_CURVE ( 'NONE', #39884, #26221, #3190, .T. ) ;
#14192=VECTOR ( 'NONE', #29109, 1000.000000000000000 ) ;
#14194=DIRECTION ( 'NONE',  ( 0.000000000000000000, 1.000000000000000000, -0.000000000000000000 ) ) ;
#14215=EDGE_CURVE ( 'NONE', #24671, #44110, #33697, .T. ) ;
#14284=FACE_OUTER_BOUND ( 'NONE', #20597, .T. ) ;
#14301=LINE ( 'NONE', #36477, #42034 ) ;
#14315=DIRECTION ( 'NONE',  ( 0.000000000000000000, 1.000000000000000000, -0.000000000000000000 ) ) ;
#14381=LINE ( 'NONE', #21576, #46143 ) ;
#14382=ORIENTED_EDGE ( 'NONE', *, *, #36587, .F. ) ;
#14405=ADVANCED_FACE ( 'NONE', ( #20891 ), #10033, .T. ) ;
#14429=VERTEX_POINT ( 'NONE', #18142 ) ;
#14432=ORIENTED_EDGE ( 'NONE', *, *, #36572, .T. ) ;
#14458=VERTEX_POINT ( 'NONE', #13717 ) ;
#14476=DIRECTION ( 'NONE',  ( 0.000000000000000000, 0.000000000000000000, -1.000000000000000000 ) ) ;
#14491=CIRCLE ( 'NONE', #7491, 0.3999999999999975797 ) ;
#14510=LINE ( 'NONE', #6922, #22868 ) ;
#14518=AXIS2_PLACEMENT_3D ( 'NONE', #47171, #28466, #35588 ) ;
#14520=EDGE_CURVE ( 'NONE', #44357, #25391, #37098, .T. ) ;
#14527=DIRECTION ( 'NONE',  ( -0.000000000000000000, -1.000000000000000000, 0.000000000000000000 ) ) ;
#14566=ORIENTED_EDGE ( 'NONE', *, *, #26458, .F. ) ;
#14602=LINE ( 'NONE', #23028, #47955 ) ;
#14612=ORIENTED_EDGE ( 'NONE', *, *, #46657, .T. ) ;
#14630=CARTESIAN_POINT ( 'NONE',  ( -50.42409385541304800, -15.80920654474410725, 63.99999999999998579 ) ) ;
#14644=ORIENTED_EDGE ( 'NONE', *, *, #37407, .T. ) ;
#14656=CARTESIAN_POINT ( 'NONE',  ( -26.42409385541305511, -8.109206544744111511, 51.75000000000000711 ) ) ;
#14670=DIRECTION ( 'NONE',  ( 0.000000000000000000, 0.000000000000000000, 1.000000000000000000 ) ) ;
#14676=ORIENTED_EDGE ( 'NONE', *, *, #23873, .T. ) ;
#14691=AXIS2_PLACEMENT_3D ( 'NONE', #25934, #3769, #38208 ) ;
#14696=CARTESIAN_POINT ( 'NONE',  ( -50.42409385541304800, -15.80920654474410725, 56.99999999999999289 ) ) ;
#14725=VECTOR ( 'NONE', #10560, 1000.000000000000000 ) ;
#14748=ORIENTED_EDGE ( 'NONE', *, *, #11769, .T. ) ;
#14751=ORIENTED_EDGE ( 'NONE', *, *, #8028, .T. ) ;
#14755=AXIS2_PLACEMENT_3D ( 'NONE', #25464, #11410, #44928 ) ;
#14831=EDGE_CURVE ( 'NONE', #9420, #11732, #44075, .T. ) ;
#14845=VECTOR ( 'NONE', #33748, 1000.000000000000000 ) ;
#14860=FACE_OUTER_BOUND ( 'NONE', #21452, .T. ) ;
#14916=AXIS2_PLACEMENT_3D ( 'NONE', #44358, #47328, #47560 ) ;
#14951=VECTOR ( 'NONE', #31915, 1000.000000000000000 ) ;
#14955=ORIENTED_EDGE ( 'NONE', *, *, #4931, .T. ) ;
#14956=ADVANCED_FACE ( 'NONE', ( #13740 ), #28785, .T. ) ;
#14967=CARTESIAN_POINT ( 'NONE',  ( -30.42409385541305156, -6.859206544744110623, 50.50000000000000000 ) ) ;
#14970=ORIENTED_EDGE ( 'NONE', *, *, #38701, .T. ) ;
#14983=ORIENTED_EDGE ( 'NONE', *, *, #26597, .T. ) ;
#14996=AXIS2_PLACEMENT_3D ( 'NONE', #31190, #19377, #669 ) ;
#15016=VECTOR ( 'NONE', #19539, 1000.000000000000000 ) ;
#15021=PLANE ( 'NONE',  #28230 ) ;
#15112=EDGE_CURVE ( 'NONE', #38065, #29761, #39079, .T. ) ;
#15116=ORIENTED_EDGE ( 'NONE', *, *, #31984, .F. ) ;
#15117=ORIENTED_EDGE ( 'NONE', *, *, #19993, .T. ) ;
#15139=DIRECTION ( 'NONE',  ( -0.000000000000000000, -1.000000000000000000, -0.000000000000000000 ) ) ;
#15151=VECTOR ( 'NONE', #31380, 1000.000000000000000 ) ;
#15159=DIRECTION ( 'NONE',  ( -0.000000000000000000, -1.000000000000000000, -0.000000000000000000 ) ) ;
#15184=ORIENTED_EDGE ( 'NONE', *, *, #33387, .F. ) ;
#15191=ORIENTED_EDGE ( 'NONE', *, *, #27519, .T. ) ;
#15267=DIRECTION ( 'NONE',  ( 1.000000000000000000, 0.000000000000000000, 0.000000000000000000 ) ) ;
#15282=DIRECTION ( 'NONE',  ( -1.000000000000000000, 0.000000000000000000, 0.000000000000000000 ) ) ;
#15285=CARTESIAN_POINT ( 'NONE',  ( -46.92409385541305511, -15.80920654474410725, 61.49999999999999289 ) ) ;
#15288=VECTOR ( 'NONE', #5801, 1000.000000000000000 ) ;
#15293=EDGE_CURVE ( 'NONE', #24724, #20623, #3773, .T. ) ;
#15345=CARTESIAN_POINT ( 'NONE',  ( -28.42409385541305511, -6.359206544744109735, 54.49999999999997158 ) ) ;
#15346=FACE_OUTER_BOUND ( 'NONE', #43681, .T. ) ;
#15394=CARTESIAN_POINT ( 'NONE',  ( -27.42409385541305511, -25.10920654474410441, 81.99999999999998579 ) ) ;
#15395=LINE ( 'NONE', #18609, #47148 ) ;
#15397=ORIENTED_EDGE ( 'NONE', *, *, #45246, .F. ) ;
#15400=ORIENTED_EDGE ( 'NONE', *, *, #10769, .T. ) ;
#15412=EDGE_LOOP ( 'NONE', ( #34231, #22287, #31036, #6822 ) ) ;
#15486=VECTOR ( 'NONE', #45581, 1000.000000000000000 ) ;
#15494=EDGE_LOOP ( 'NONE', ( #31623, #37571, #13676, #24271, #4395 ) ) ;
#15510=DIRECTION ( 'NONE',  ( -0.000000000000000000, -1.000000000000000000, -0.000000000000000000 ) ) ;
#15514=ORIENTED_EDGE ( 'NONE', *, *, #36337, .T. ) ;
#15533=( LENGTH_UNIT ( ) NAMED_UNIT ( * ) SI_UNIT ( .MILLI., .METRE. ) );
#15541=ORIENTED_EDGE ( 'NONE', *, *, #30697, .F. ) ;
#15542=ORIENTED_EDGE ( 'NONE', *, *, #38444, .F. ) ;
#15554=CIRCLE ( 'NONE', #22681, 2.000000000000001776 ) ;
#15574=LINE ( 'NONE', #38479, #32926 ) ;
#15595=VECTOR ( 'NONE', #35571, 1000.000000000000000 ) ;
#15657=DIRECTION ( 'NONE',  ( 0.000000000000000000, 0.000000000000000000, 1.000000000000000000 ) ) ;
#15660=LINE ( 'NONE', #19612, #2743 ) ;
#15665=ORIENTED_EDGE ( 'NONE', *, *, #45246, .T. ) ;
#15695=ORIENTED_EDGE ( 'NONE', *, *, #25095, .T. ) ;
#15705=EDGE_CURVE ( 'NONE', #31278, #41929, #8525, .T. ) ;
#15714=AXIS2_PLACEMENT_3D ( 'NONE', #19063, #18309, #30165 ) ;
#15735=EDGE_CURVE ( 'NONE', #3842, #4984, #8451, .T. ) ;
#15737=AXIS2_PLACEMENT_3D ( 'NONE', #33572, #33834, #130 ) ;
#15769=CIRCLE ( 'NONE', #4794, 2.000000000000001776 ) ;
#15776=CARTESIAN_POINT ( 'NONE',  ( -18.92409385541305511, -14.80920654474410547, 48.99999999999997868 ) ) ;
#15786=CARTESIAN_POINT ( 'NONE',  ( -6.424093855413055110, -6.859206544744110623, 47.99999999999998579 ) ) ;
#15787=LINE ( 'NONE', #20217, #11187 ) ;
#15789=ORIENTED_EDGE ( 'NONE', *, *, #44457, .F. ) ;
#15808=DIRECTION ( 'NONE',  ( 0.000000000000000000, 1.000000000000000000, -0.000000000000000000 ) ) ;
#15823=CARTESIAN_POINT ( 'NONE',  ( -8.424093855413060439, -6.359206544744109735, 47.99999999999998579 ) ) ;
#15865=ORIENTED_EDGE ( 'NONE', *, *, #8442, .T. ) ;
#15871=FACE_OUTER_BOUND ( 'NONE', #44811, .T. ) ;
#15915=ORIENTED_EDGE ( 'NONE', *, *, #1713, .F. ) ;
#15925=DIRECTION ( 'NONE',  ( 0.000000000000000000, 0.000000000000000000, -1.000000000000000000 ) ) ;
#15948=DIRECTION ( 'NONE',  ( 0.000000000000000000, 0.000000000000000000, 1.000000000000000000 ) ) ;
#16004=DIRECTION ( 'NONE',  ( -1.000000000000000000, 0.000000000000000000, 0.000000000000000000 ) ) ;
#16005=CARTESIAN_POINT ( 'NONE',  ( -27.42409385541305511, -25.10920654474410441, 54.99999999999997868 ) ) ;
#16023=EDGE_CURVE ( 'NONE', #20442, #28963, #3853, .T. ) ;
#16027=CARTESIAN_POINT ( 'NONE',  ( -30.42409385541305156, -6.859206544744110623, 52.99999999999997158 ) ) ;
#16097=CARTESIAN_POINT ( 'NONE',  ( -40.64308517176574753, -25.10920654474410441, 77.24806946917840378 ) ) ;
#16123=LINE ( 'NONE', #15394, #19590 ) ;
#16129=ORIENTED_EDGE ( 'NONE', *, *, #10303, .T. ) ;
#16161=DIRECTION ( 'NONE',  ( 1.000000000000000000, 0.000000000000000000, 0.000000000000000000 ) ) ;
#16168=FACE_OUTER_BOUND ( 'NONE', #29755, .T. ) ;
#16195=DIRECTION ( 'NONE',  ( 1.000000000000000000, -0.000000000000000000, 0.000000000000000000 ) ) ;
#16199=AXIS2_PLACEMENT_3D ( 'NONE', #19562, #26715, #20293 ) ;
#16224=AXIS2_PLACEMENT_3D ( 'NONE', #37397, #33458, #2947 ) ;
#16227=DIRECTION ( 'NONE',  ( 1.000000000000000000, 0.000000000000000000, -9.637352644315596475E-17 ) ) ;
#16241=CARTESIAN_POINT ( 'NONE',  ( -48.42409385541304800, -27.10920654474410796, 47.99999999999998579 ) ) ;
#16257=FILL_AREA_STYLE_COLOUR ( '', #38407 ) ;
#16275=EDGE_CURVE ( 'NONE', #29613, #43808, #9252, .T. ) ;
#16306=DIRECTION ( 'NONE',  ( -0.000000000000000000, -1.000000000000000000, -0.000000000000000000 ) ) ;
#16322=DIRECTION ( 'NONE',  ( 0.000000000000000000, 0.000000000000000000, 1.000000000000000000 ) ) ;
#16341=VERTEX_POINT ( 'NONE', #35090 ) ;
#16399=LINE ( 'NONE', #31428, #16581 ) ;
#16409=AXIS2_PLACEMENT_3D ( 'NONE', #38171, #15510, #42131 ) ;
#16411=CARTESIAN_POINT ( 'NONE',  ( -50.42409385541304800, -15.80920654474410725, 74.99999999999998579 ) ) ;
#16412=ADVANCED_FACE ( 'NONE', ( #20814 ), #2584, .F. ) ;
#16438=ADVANCED_FACE ( 'NONE', ( #6282 ), #13879, .F. ) ;
#16448=FACE_OUTER_BOUND ( 'NONE', #45108, .T. ) ;
#16459=ORIENTED_EDGE ( 'NONE', *, *, #26182, .T. ) ;
#16516=CARTESIAN_POINT ( 'NONE',  ( -20.92409385541305511, -10.10920654474410618, 81.49999999999998579 ) ) ;
#16531=EDGE_LOOP ( 'NONE', ( #21461, #11898, #29779, #47292 ) ) ;
#16532=LINE ( 'NONE', #12610, #17848 ) ;
#16547=ORIENTED_EDGE ( 'NONE', *, *, #47622, .F. ) ;
#16558=DIRECTION ( 'NONE',  ( 2.168404344971008375E-16, 0.000000000000000000, -1.000000000000000000 ) ) ;
#16581=VECTOR ( 'NONE', #2115, 1000.000000000000000 ) ;
#16599=CARTESIAN_POINT ( 'NONE',  ( -6.424093855413058662, -6.859206544744110623, 52.99999999999998579 ) ) ;
#16600=CARTESIAN_POINT ( 'NONE',  ( -27.42409385541305511, -25.10920654474410441, 78.99999999999998579 ) ) ;
#16616=AXIS2_PLACEMENT_3D ( 'NONE', #40605, #44101, #33446 ) ;
#16628=ORIENTED_EDGE ( 'NONE', *, *, #20874, .F. ) ;
#16684=LINE ( 'NONE', #43043, #19413 ) ;
#16699=DIRECTION ( 'NONE',  ( 0.000000000000000000, 0.000000000000000000, 1.000000000000000000 ) ) ;
#16739=PLANE ( 'NONE',  #27120 ) ;
#16754=EDGE_CURVE ( 'NONE', #42423, #42114, #29789, .T. ) ;
#16757=CARTESIAN_POINT ( 'NONE',  ( -13.92409385541305511, -10.10920654474410618, 81.99999999999998579 ) ) ;
#16777=EDGE_LOOP ( 'NONE', ( #16628, #23982, #20269, #20501 ) ) ;
#16780=DIRECTION ( 'NONE',  ( 0.000000000000000000, 0.000000000000000000, 1.000000000000000000 ) ) ;
#16782=DIRECTION ( 'NONE',  ( 1.000000000000000000, -0.000000000000000000, 2.081668171172170091E-15 ) ) ;
#16786=DIRECTION ( 'NONE',  ( 0.000000000000000000, 0.000000000000000000, -1.000000000000000000 ) ) ;
#16806=CARTESIAN_POINT ( 'NONE',  ( -4.424093855413056886, -25.10920654474410441, 79.99999999999998579 ) ) ;
#16811=AXIS2_PLACEMENT_3D ( 'NONE', #23964, #12860, #27885 ) ;
#16827=CARTESIAN_POINT ( 'NONE',  ( -28.42409385541305511, -6.859206544744110623, 54.99999999999996447 ) ) ;
#16842=CARTESIAN_POINT ( 'NONE',  ( -26.42409385541305511, -8.109206544744111511, 50.50000000000000000 ) ) ;
#16847=LINE ( 'NONE', #31886, #23460 ) ;
#16871=CIRCLE ( 'NONE', #33377, 1.500000000000008216 ) ;
#16921=DIRECTION ( 'NONE',  ( 0.000000000000000000, 0.000000000000000000, 1.000000000000000000 ) ) ;
#16970=LINE ( 'NONE', #47029, #18385 ) ;
#16983=CARTESIAN_POINT ( 'NONE',  ( -8.424093855413094190, -25.10920654474410441, 64.00000000000002842 ) ) ;
#17036=DIRECTION ( 'NONE',  ( 0.000000000000000000, 0.000000000000000000, 1.000000000000000000 ) ) ;
#17063=DIRECTION ( 'NONE',  ( -9.637352644315596475E-17, 0.000000000000000000, -1.000000000000000000 ) ) ;
#17081=ORIENTED_EDGE ( 'NONE', *, *, #46969, .F. ) ;
#17095=ADVANCED_FACE ( 'NONE', ( #36714 ), #5984, .F. ) ;
#17096=DIRECTION ( 'NONE',  ( -1.000000000000000000, 0.000000000000000000, 0.000000000000000000 ) ) ;
#17123=DIRECTION ( 'NONE',  ( 0.000000000000000000, 0.000000000000000000, -1.000000000000000000 ) ) ;
#17124=DIRECTION ( 'NONE',  ( 0.000000000000000000, 0.000000000000000000, 1.000000000000000000 ) ) ;
#17144=VERTEX_POINT ( 'NONE', #32801 ) ;
#17173=CARTESIAN_POINT ( 'NONE',  ( -6.424093855413058662, -6.859206544744110623, 54.99999999999999289 ) ) ;
#17204=CARTESIAN_POINT ( 'NONE',  ( -30.42409385541305156, -25.10920654474410441, 52.99999999999997158 ) ) ;
#17215=CARTESIAN_POINT ( 'NONE',  ( -27.42409385541305511, -6.359206544744109735, 63.99999999999998579 ) ) ;
#17235=CARTESIAN_POINT ( 'NONE',  ( -43.17409385541305511, -15.80920654474410725, 56.99999999999999289 ) ) ;
#17318=DIRECTION ( 'NONE',  ( -0.000000000000000000, -1.000000000000000000, -0.000000000000000000 ) ) ;
#17330=CIRCLE ( 'NONE', #40927, 1.250000000000001110 ) ;
#17332=DIRECTION ( 'NONE',  ( 1.000000000000000000, 0.000000000000000000, 0.000000000000000000 ) ) ;
#17336=CARTESIAN_POINT ( 'NONE',  ( -26.92409385541305511, -6.859206544744110623, 52.99999999999997158 ) ) ;
#17363=ORIENTED_EDGE ( 'NONE', *, *, #26119, .T. ) ;
#17376=EDGE_CURVE ( 'NONE', #34652, #23071, #37432, .T. ) ;
#17385=ADVANCED_FACE ( 'NONE', ( #23420 ), #19468, .T. ) ;
#17413=ORIENTED_EDGE ( 'NONE', *, *, #46969, .T. ) ;
#17425=VERTEX_POINT ( 'NONE', #7930 ) ;
#17451=CARTESIAN_POINT ( 'NONE',  ( -8.424093855413094190, -15.80920654474410725, 64.00000000000002842 ) ) ;
#17464=CARTESIAN_POINT ( 'NONE',  ( -41.15852941833841783, -27.10920654474410796, 54.99999999999997868 ) ) ;
#17465=VERTEX_POINT ( 'NONE', #9130 ) ;
#17494=EDGE_CURVE ( 'NONE', #38652, #44500, #18816, .T. ) ;
#17525=LINE ( 'NONE', #10151, #27160 ) ;
#17527=VERTEX_POINT ( 'NONE', #13273 ) ;
#17534=DIRECTION ( 'NONE',  ( 0.000000000000000000, 0.000000000000000000, 1.000000000000000000 ) ) ;
#17537=VERTEX_POINT ( 'NONE', #46566 ) ;
#17590=DIRECTION ( 'NONE',  ( 0.000000000000000000, 1.000000000000000000, 0.000000000000000000 ) ) ;
#17597=DIRECTION ( 'NONE',  ( 0.000000000000000000, -1.000000000000000000, 0.000000000000000000 ) ) ;
#17620=VERTEX_POINT ( 'NONE', #7132 ) ;
#17639=DIRECTION ( 'NONE',  ( -0.000000000000000000, -0.000000000000000000, 1.000000000000000000 ) ) ;
#17666=FACE_OUTER_BOUND ( 'NONE', #42382, .T. ) ;
#17715=PLANE ( 'NONE',  #28767 ) ;
#17766=CARTESIAN_POINT ( 'NONE',  ( -35.32409385541306079, -8.109206544744111511, 49.44999999999998863 ) ) ;
#17796=ADVANCED_FACE ( 'NONE', ( #27775 ), #1424, .T. ) ;
#17801=CARTESIAN_POINT ( 'NONE',  ( -26.42409385541305511, -6.359206544744109735, 47.99999999999997868 ) ) ;
#17805=CARTESIAN_POINT ( 'NONE',  ( -17.42409385541305511, -14.80920654474410725, 79.00000000000000000 ) ) ;
#17810=CIRCLE ( 'NONE', #24900, 1.250000000000001110 ) ;
#17818=VECTOR ( 'NONE', #37327, 1000.000000000000000 ) ;
#17827=ORIENTED_EDGE ( 'NONE', *, *, #10316, .T. ) ;
#17835=DIRECTION ( 'NONE',  ( -1.000000000000000000, 0.000000000000000000, -1.927470528863119295E-16 ) ) ;
#17840=VECTOR ( 'NONE', #6826, 1000.000000000000000 ) ;
#17848=VECTOR ( 'NONE', #5228, 1000.000000000000000 ) ;
#17850=DIRECTION ( 'NONE',  ( -2.168404344971008375E-16, -0.000000000000000000, 1.000000000000000000 ) ) ;
#17862=DIRECTION ( 'NONE',  ( 0.000000000000000000, 0.000000000000000000, 1.000000000000000000 ) ) ;
#17863=ORIENTED_EDGE ( 'NONE', *, *, #6547, .T. ) ;
#17896=DIRECTION ( 'NONE',  ( 0.000000000000000000, 0.000000000000000000, 1.000000000000000000 ) ) ;
#17907=CIRCLE ( 'NONE', #17945, 1.999999999999994893 ) ;
#17934=LINE ( 'NONE', #13988, #27083 ) ;
#17938=EDGE_LOOP ( 'NONE', ( #45583, #40828, #46602, #37378 ) ) ;
#17941=AXIS2_PLACEMENT_3D ( 'NONE', #11584, #39137, #16227 ) ;
#17945=AXIS2_PLACEMENT_3D ( 'NONE', #12991, #28019, #9323 ) ;
#17976=CIRCLE ( 'NONE', #3854, 1.000000000000000888 ) ;
#17977=ORIENTED_EDGE ( 'NONE', *, *, #3619, .F. ) ;
#18001=ORIENTED_EDGE ( 'NONE', *, *, #14831, .T. ) ;
#18064=AXIS2_PLACEMENT_3D ( 'NONE', #1428, #24337, #16921 ) ;
#18065=CARTESIAN_POINT ( 'NONE',  ( -18.92409385541305511, -14.80920654474410547, 52.21286476528345588 ) ) ;
#18068=CARTESIAN_POINT ( 'NONE',  ( -6.424093855413055110, -27.10920654474410796, 79.99999999999998579 ) ) ;
#18092=ORIENTED_EDGE ( 'NONE', *, *, #43249, .T. ) ;
#18096=CARTESIAN_POINT ( 'NONE',  ( -33.52409385541305653, -25.10920654474410441, 52.29999999999998295 ) ) ;
#18119=ORIENTED_EDGE ( 'NONE', *, *, #48610, .F. ) ;
#18124=DIRECTION ( 'NONE',  ( 1.000000000000000000, 0.000000000000000000, 0.000000000000000000 ) ) ;
#18142=CARTESIAN_POINT ( 'NONE',  ( -15.92409385541305333, -15.80920654474410725, 47.99999999999998579 ) ) ;
#18186=CARTESIAN_POINT ( 'NONE',  ( -33.52409385541305653, -2.423472813913224222, 48.79999999999998295 ) ) ;
#18190=EDGE_LOOP ( 'NONE', ( #14566, #650, #39064, #9856 ) ) ;
#18266=CARTESIAN_POINT ( 'NONE',  ( -28.42409385541305511, -6.359206544744109735, 52.99999999999997158 ) ) ;
#18309=DIRECTION ( 'NONE',  ( -1.000000000000000000, 0.000000000000000000, 8.260587980841940012E-17 ) ) ;
#18321=EDGE_LOOP ( 'NONE', ( #46817, #32841, #14382, #35919, #18964 ) ) ;
#18358=CARTESIAN_POINT ( 'NONE',  ( -6.424093855413055110, -25.10920654474410441, 79.99999999999998579 ) ) ;
#18364=ORIENTED_EDGE ( 'NONE', *, *, #39608, .T. ) ;
#18385=VECTOR ( 'NONE', #32014, 1000.000000000000114 ) ;
#18396=ORIENTED_EDGE ( 'NONE', *, *, #2103, .F. ) ;
#18406=VERTEX_POINT ( 'NONE', #31784 ) ;
#18416=AXIS2_PLACEMENT_3D ( 'NONE', #1180, #35870, #46505 ) ;
#18440=ADVANCED_FACE ( 'NONE', ( #39652 ), #5923, .F. ) ;
#18450=CIRCLE ( 'NONE', #10596, 1.999999999999994893 ) ;
#18459=ADVANCED_FACE ( 'NONE', ( #44563 ), #6165, .T. ) ;
#18479=ORIENTED_EDGE ( 'NONE', *, *, #35978, .F. ) ;
#18519=CIRCLE ( 'NONE', #2011, 2.000000000000001776 ) ;
#18531=EDGE_CURVE ( 'NONE', #14429, #13748, #42453, .T. ) ;
#18556=DIRECTION ( 'NONE',  ( 0.000000000000000000, 0.000000000000000000, 1.000000000000000000 ) ) ;
#18559=ORIENTED_EDGE ( 'NONE', *, *, #42892, .T. ) ;
#18579=CIRCLE ( 'NONE', #33550, 0.5000000000000004441 ) ;
#18580=AXIS2_PLACEMENT_3D ( 'NONE', #5708, #32039, #5936 ) ;
#18585=CARTESIAN_POINT ( 'NONE',  ( -17.90106345612152694, -14.65920654474411045, 52.21286476528345588 ) ) ;
#18609=CARTESIAN_POINT ( 'NONE',  ( -7.424093855413048892, -25.10920654474410441, 56.99999999999997868 ) ) ;
#18650=EDGE_CURVE ( 'NONE', #28963, #26610, #12520, .T. ) ;
#18655=AXIS2_PLACEMENT_3D ( 'NONE', #9816, #21617, #47712 ) ;
#18656=VECTOR ( 'NONE', #19029, 1000.000000000000000 ) ;
#18664=ORIENTED_EDGE ( 'NONE', *, *, #2839, .T. ) ;
#18691=EDGE_CURVE ( 'NONE', #26808, #26269, #42813, .T. ) ;
#18771=ORIENTED_EDGE ( 'NONE', *, *, #40228, .T. ) ;
#18780=AXIS2_PLACEMENT_3D ( 'NONE', #39692, #21227, #43643 ) ;
#18809=ORIENTED_EDGE ( 'NONE', *, *, #1937, .F. ) ;
#18810=CARTESIAN_POINT ( 'NONE',  ( -27.42409385541305156, -25.10920654474410441, 47.99999999999997868 ) ) ;
#18816=CIRCLE ( 'NONE', #43972, 2.000000000000001776 ) ;
#18831=EDGE_CURVE ( 'NONE', #41762, #21252, #7086, .T. ) ;
#18833=LINE ( 'NONE', #38021, #46538 ) ;
#18891=VERTEX_POINT ( 'NONE', #11495 ) ;
#18899=CARTESIAN_POINT ( 'NONE',  ( -17.42409385541305511, -14.80920654474410725, 81.99999999999998579 ) ) ;
#18900=EDGE_CURVE ( 'NONE', #39233, #24954, #32250, .T. ) ;
#18936=DIRECTION ( 'NONE',  ( -1.000000000000000000, 0.000000000000000000, 8.260587980841940012E-17 ) ) ;
#18942=DIRECTION ( 'NONE',  ( 2.181982678098338148E-16, 0.000000000000000000, -1.000000000000000000 ) ) ;
#18964=ORIENTED_EDGE ( 'NONE', *, *, #96, .F. ) ;
#18976=CIRCLE ( 'NONE', #26865, 1.250000000000001110 ) ;
#18985=PLANE ( 'NONE',  #34523 ) ;
#18989=AXIS2_PLACEMENT_3D ( 'NONE', #27208, #30918, #20566 ) ;
#19009=AXIS2_PLACEMENT_3D ( 'NONE', #47340, #2511, #16786 ) ;
#19029=DIRECTION ( 'NONE',  ( 1.927470528863119542E-16, 0.000000000000000000, -1.000000000000000000 ) ) ;
#19063=CARTESIAN_POINT ( 'NONE',  ( -27.42409385541305511, -10.60920654474410618, 81.49999999999998579 ) ) ;
#19084=CARTESIAN_POINT ( 'NONE',  ( -27.42409385541305511, -27.10920654474410796, 63.99999999999998579 ) ) ;
#19098=CARTESIAN_POINT ( 'NONE',  ( -33.95962776134579286, -8.109206544744111511, 51.75000000000000711 ) ) ;
#19118=DIRECTION ( 'NONE',  ( 1.000000000000000000, 0.000000000000000000, 0.000000000000000000 ) ) ;
#19124=ORIENTED_EDGE ( 'NONE', *, *, #42475, .T. ) ;
#19129=CARTESIAN_POINT ( 'NONE',  ( -4.424093855413056886, -8.109206544744111511, 50.49999999999999289 ) ) ;
#19146=ORIENTED_EDGE ( 'NONE', *, *, #24903, .T. ) ;
#19204=AXIS2_PLACEMENT_3D ( 'NONE', #31544, #38685, #1248 ) ;
#19217=EDGE_CURVE ( 'NONE', #41525, #44500, #14602, .T. ) ;
#19257=DIRECTION ( 'NONE',  ( 1.000000000000000000, -0.000000000000000000, -2.406186529621654511E-16 ) ) ;
#19296=CARTESIAN_POINT ( 'NONE',  ( -8.424093855413053333, -15.80920654474410725, 47.99999999999998579 ) ) ;
#19300=EDGE_CURVE ( 'NONE', #24671, #16341, #34626, .T. ) ;
#19323=DIRECTION ( 'NONE',  ( 0.000000000000000000, 0.000000000000000000, 1.000000000000000000 ) ) ;
#19377=DIRECTION ( 'NONE',  ( 1.927470528863119542E-16, 0.000000000000000000, -1.000000000000000000 ) ) ;
#19383=CIRCLE ( 'NONE', #27257, 0.5000000000000004441 ) ;
#19397=DIRECTION ( 'NONE',  ( 0.000000000000000000, 0.000000000000000000, 1.000000000000000000 ) ) ;
#19407=EDGE_LOOP ( 'NONE', ( #410, #36724, #21326, #44353 ) ) ;
#19413=VECTOR ( 'NONE', #9321, 1000.000000000000000 ) ;
#19421=CIRCLE ( 'NONE', #4520, 1.999999999999994893 ) ;
#19432=( NAMED_UNIT ( * ) PLANE_ANGLE_UNIT ( ) SI_UNIT ( $, .RADIAN. ) );
#19439=CARTESIAN_POINT ( 'NONE',  ( -4.924093855413050669, -6.859206544744110623, 52.99999999999998579 ) ) ;
#19443=ORIENTED_EDGE ( 'NONE', *, *, #45204, .T. ) ;
#19450=AXIS2_PLACEMENT_3D ( 'NONE', #35495, #15808, #23465 ) ;
#19453=ORIENTED_EDGE ( 'NONE', *, *, #36771, .T. ) ;
#19468=CYLINDRICAL_SURFACE ( 'NONE', #16409, 2.000000000000001776 ) ;
#19488=FILL_AREA_STYLE ('',( #16257 ) ) ;
#19513=EDGE_LOOP ( 'NONE', ( #45861, #22293, #42933, #14432, #34874, #12932, #15397, #14676 ) ) ;
#19520=DIRECTION ( 'NONE',  ( 1.000000000000000000, 0.000000000000000000, 0.000000000000000000 ) ) ;
#19539=DIRECTION ( 'NONE',  ( -0.000000000000000000, -1.000000000000000000, -0.000000000000000000 ) ) ;
#19562=CARTESIAN_POINT ( 'NONE',  ( -20.92409385541305511, -10.10920654474410618, 80.49999999999998579 ) ) ;
#19564=CARTESIAN_POINT ( 'NONE',  ( -41.15852941833841783, -25.10920654474410441, 54.99999999999997868 ) ) ;
#19574=ORIENTED_EDGE ( 'NONE', *, *, #1678, .T. ) ;
#19586=CYLINDRICAL_SURFACE ( 'NONE', #33908, 1.250000000000001110 ) ;
#19590=VECTOR ( 'NONE', #31168, 1000.000000000000000 ) ;
#19612=CARTESIAN_POINT ( 'NONE',  ( -33.95962776134579286, -8.109206544744111511, 49.25000000000000000 ) ) ;
#19615=DIRECTION ( 'NONE',  ( 0.000000000000000000, 0.000000000000000000, 1.000000000000000000 ) ) ;
#19619=ORIENTED_EDGE ( 'NONE', *, *, #13070, .F. ) ;
#19633=CARTESIAN_POINT ( 'NONE',  ( -8.424093855413071097, -25.10920654474410441, 52.99999999999997868 ) ) ;
#19655=DIRECTION ( 'NONE',  ( -0.000000000000000000, -1.000000000000000000, 9.912705577010318647E-16 ) ) ;
#19690=VERTEX_POINT ( 'NONE', #39111 ) ;
#19697=AXIS2_PLACEMENT_3D ( 'NONE', #39449, #31816, #13561 ) ;
#19775=CYLINDRICAL_SURFACE ( 'NONE', #3950, 0.5000000000000004441 ) ;
#19786=DIRECTION ( 'NONE',  ( 0.000000000000000000, 0.000000000000000000, 1.000000000000000000 ) ) ;
#19792=AXIS2_PLACEMENT_3D ( 'NONE', #42054, #45993, #19397 ) ;
#19815=DIRECTION ( 'NONE',  ( 0.000000000000000000, 1.000000000000000000, 0.000000000000000000 ) ) ;
#19832=DIRECTION ( 'NONE',  ( -0.000000000000000000, -1.000000000000000000, -0.000000000000000000 ) ) ;
#19847=DIRECTION ( 'NONE',  ( -1.000000000000000000, 0.000000000000000000, -2.181982678098338148E-16 ) ) ;
#19854=EDGE_LOOP ( 'NONE', ( #41348, #35706, #18001, #36162, #14955, #40301, #27692, #1102 ) ) ;
#19855=CARTESIAN_POINT ( 'NONE',  ( -27.42409385541305511, -25.10920654474410441, 48.99999999999997868 ) ) ;
#19886=CARTESIAN_POINT ( 'NONE',  ( -17.42409385541305511, -14.80920654474410725, 48.99999999999997868 ) ) ;
#19962=CARTESIAN_POINT ( 'NONE',  ( -30.42409385541305156, -6.359206544744109735, 47.99999999999997868 ) ) ;
#19972=VERTEX_POINT ( 'NONE', #12717 ) ;
#19978=LINE ( 'NONE', #8661, #12905 ) ;
#19993=EDGE_CURVE ( 'NONE', #41987, #37795, #39049, .T. ) ;
#20026=CARTESIAN_POINT ( 'NONE',  ( -27.42409385541305511, -15.80920654474410725, 63.99999999999998579 ) ) ;
#20027=DIRECTION ( 'NONE',  ( 1.000000000000000000, -0.000000000000000000, 0.000000000000000000 ) ) ;
#20044=DIRECTION ( 'NONE',  ( 0.000000000000000000, 0.000000000000000000, -1.000000000000000000 ) ) ;
#20063=ORIENTED_EDGE ( 'NONE', *, *, #10769, .F. ) ;
#20087=ORIENTED_EDGE ( 'NONE', *, *, #24945, .T. ) ;
#20093=VERTEX_POINT ( 'NONE', #11915 ) ;
#20101=VERTEX_POINT ( 'NONE', #30150 ) ;
#20113=DIRECTION ( 'NONE',  ( 1.927470528863119542E-16, 0.000000000000000000, -1.000000000000000000 ) ) ;
#20134=CARTESIAN_POINT ( 'NONE',  ( -38.65852941833841783, -25.10920654474410441, 78.99999999999998579 ) ) ;
#20146=VERTEX_POINT ( 'NONE', #45175 ) ;
#20164=CARTESIAN_POINT ( 'NONE',  ( -35.32409385541306079, -6.359206544744109735, 51.54999999999998295 ) ) ;
#20166=CARTESIAN_POINT ( 'NONE',  ( -4.424093855413049781, -25.10920654474410441, 52.99999999999998579 ) ) ;
#20180=EDGE_LOOP ( 'NONE', ( #11984, #24659, #23782, #3538 ) ) ;
#20183=VECTOR ( 'NONE', #44830, 1000.000000000000000 ) ;
#20204=CARTESIAN_POINT ( 'NONE',  ( -35.32409385541306079, -8.109206544744111511, 51.54999999999998295 ) ) ;
#20217=CARTESIAN_POINT ( 'NONE',  ( -50.42409385541304800, -25.10920654474410441, 63.99999999999998579 ) ) ;
#20266=EDGE_CURVE ( 'NONE', #33080, #20101, #9680, .T. ) ;
#20269=ORIENTED_EDGE ( 'NONE', *, *, #22508, .T. ) ;
#20270=FACE_BOUND ( 'NONE', #43201, .T. ) ;
#20289=FACE_OUTER_BOUND ( 'NONE', #28911, .T. ) ;
#20293=DIRECTION ( 'NONE',  ( 0.000000000000000000, 0.000000000000000000, -1.000000000000000000 ) ) ;
#20296=VECTOR ( 'NONE', #19655, 1000.000000000000000 ) ;
#20306=VECTOR ( 'NONE', #44505, 1000.000000000000000 ) ;
#20328=DIRECTION ( 'NONE',  ( 0.000000000000000000, 0.000000000000000000, -1.000000000000000000 ) ) ;
#20420=VECTOR ( 'NONE', #7199, 1000.000000000000000 ) ;
#20426=CYLINDRICAL_SURFACE ( 'NONE', #33093, 1.250000000000007994 ) ;
#20442=VERTEX_POINT ( 'NONE', #8090 ) ;
#20476=CIRCLE ( 'NONE', #19697, 1.250000000000001110 ) ;
#20501=ORIENTED_EDGE ( 'NONE', *, *, #48546, .F. ) ;
#20502=CARTESIAN_POINT ( 'NONE',  ( -8.424093855413094190, -6.359206544744109735, 64.00000000000002842 ) ) ;
#20524=CIRCLE ( 'NONE', #41745, 1.999999999999994893 ) ;
#20548=AXIS2_PLACEMENT_3D ( 'NONE', #21884, #29516, #32488 ) ;
#20566=DIRECTION ( 'NONE',  ( 0.000000000000000000, 0.000000000000000000, 1.000000000000000000 ) ) ;
#20587=EDGE_CURVE ( 'NONE', #39291, #7384, #42554, .T. ) ;
#20597=EDGE_LOOP ( 'NONE', ( #18396, #30435, #33702, #36291 ) ) ;
#20623=VERTEX_POINT ( 'NONE', #10490 ) ;
#20631=EDGE_CURVE ( 'NONE', #44357, #42725, #35466, .T. ) ;
#20653=ORIENTED_EDGE ( 'NONE', *, *, #47403, .T. ) ;
#20700=CARTESIAN_POINT ( 'NONE',  ( -27.42409385541305156, -14.65920654474411045, 48.99999999999997868 ) ) ;
#20702=ORIENTED_EDGE ( 'NONE', *, *, #40228, .F. ) ;
#20714=ORIENTED_EDGE ( 'NONE', *, *, #15735, .T. ) ;
#20734=ORIENTED_EDGE ( 'NONE', *, *, #31880, .F. ) ;
#20752=DIRECTION ( 'NONE',  ( -0.000000000000000000, -1.000000000000000000, 0.000000000000000000 ) ) ;
#20766=AXIS2_PLACEMENT_3D ( 'NONE', #8050, #34349, #635 ) ;
#20793=CARTESIAN_POINT ( 'NONE',  ( -20.92409385541305511, -10.60920654474410618, 79.49999999999998579 ) ) ;
#20801=DIRECTION ( 'NONE',  ( 0.000000000000000000, 0.000000000000000000, -1.000000000000000000 ) ) ;
#20814=FACE_OUTER_BOUND ( 'NONE', #4647, .T. ) ;
#20834=CIRCLE ( 'NONE', #40469, 2.000000000000001776 ) ;
#20846=CARTESIAN_POINT ( 'NONE',  ( -27.42409385541305511, -15.80920654474410725, 48.99999999999997868 ) ) ;
#20874=EDGE_CURVE ( 'NONE', #4687, #34669, #34577, .T. ) ;
#20891=FACE_OUTER_BOUND ( 'NONE', #36589, .T. ) ;
#20929=VECTOR ( 'NONE', #13026, 1000.000000000000000 ) ;
#20944=CARTESIAN_POINT ( 'NONE',  ( -30.42409385541305156, -6.359206544744109735, 63.99999999999998579 ) ) ;
#20948=ADVANCED_FACE ( 'NONE', ( #5537 ), #10197, .F. ) ;
#20970=EDGE_LOOP ( 'NONE', ( #5808, #26537, #26508, #8957 ) ) ;
#20976=ORIENTED_EDGE ( 'NONE', *, *, #10002, .T. ) ;
#20983=VERTEX_POINT ( 'NONE', #16827 ) ;
#20994=CARTESIAN_POINT ( 'NONE',  ( -46.92409385541305511, -15.80920654474410725, 61.49999999999999289 ) ) ;
#21010=CARTESIAN_POINT ( 'NONE',  ( -35.32409385541306079, -6.359206544744109735, 49.44999999999998863 ) ) ;
#21027=DIRECTION ( 'NONE',  ( 1.000000000000000000, 0.000000000000000000, 0.000000000000000000 ) ) ;
#21034=DIRECTION ( 'NONE',  ( 1.927470528863119542E-16, 0.000000000000000000, -1.000000000000000000 ) ) ;
#21096=CIRCLE ( 'NONE', #13305, 0.5000000000000004441 ) ;
#21151=AXIS2_PLACEMENT_3D ( 'NONE', #22431, #29830, #33001 ) ;
#21157=DIRECTION ( 'NONE',  ( -1.000000000000000000, 0.000000000000000000, 9.637352644315596475E-17 ) ) ;
#21182=ORIENTED_EDGE ( 'NONE', *, *, #28709, .T. ) ;
#21209=CARTESIAN_POINT ( 'NONE',  ( -30.42409385541305156, -8.109206544744111511, 50.50000000000000000 ) ) ;
#21214=VECTOR ( 'NONE', #1855, 1000.000000000000000 ) ;
#21227=DIRECTION ( 'NONE',  ( 0.000000000000000000, -0.000000000000000000, 1.000000000000000000 ) ) ;
#21229=DIRECTION ( 'NONE',  ( 1.927470528863119542E-16, 0.000000000000000000, -1.000000000000000000 ) ) ;
#21252=VERTEX_POINT ( 'NONE', #43389 ) ;
#21286=EDGE_CURVE ( 'NONE', #24954, #26610, #6411, .T. ) ;
#21293=AXIS2_PLACEMENT_3D ( 'NONE', #12018, #27754, #38333 ) ;
#21295=CARTESIAN_POINT ( 'NONE',  ( -26.92409385541305511, -6.359206544744109735, 52.99999999999997158 ) ) ;
#21309=DIRECTION ( 'NONE',  ( 0.000000000000000000, 0.000000000000000000, -1.000000000000000000 ) ) ;
#21325=EDGE_LOOP ( 'NONE', ( #44783, #7812, #12113, #18771 ) ) ;
#21326=ORIENTED_EDGE ( 'NONE', *, *, #20266, .T. ) ;
#21328=PLANE ( 'NONE',  #9524 ) ;
#21333=EDGE_CURVE ( 'NONE', #112, #20093, #23605, .T. ) ;
#21353=AXIS2_PLACEMENT_3D ( 'NONE', #10123, #21457, #2722 ) ;
#21372=CIRCLE ( 'NONE', #25304, 2.000000000000001776 ) ;
#21402=LINE ( 'NONE', #47974, #47949 ) ;
#21440=EDGE_CURVE ( 'NONE', #31120, #38065, #12486, .T. ) ;
#21452=EDGE_LOOP ( 'NONE', ( #36436, #6400, #43974, #39539 ) ) ;
#21457=DIRECTION ( 'NONE',  ( 1.000000000000000000, 0.000000000000000000, -2.406186529621654018E-16 ) ) ;
#21460=CARTESIAN_POINT ( 'NONE',  ( -28.42409385541305511, -6.859206544744110623, 47.99999999999997868 ) ) ;
#21461=ORIENTED_EDGE ( 'NONE', *, *, #26182, .F. ) ;
#21519=EDGE_CURVE ( 'NONE', #17620, #9150, #2843, .T. ) ;
#21563=EDGE_CURVE ( 'NONE', #11264, #25709, #28718, .T. ) ;
#21575=ORIENTED_EDGE ( 'NONE', *, *, #35314, .T. ) ;
#21576=CARTESIAN_POINT ( 'NONE',  ( -4.424093855413053333, -6.859206544744110623, 63.99999999999998579 ) ) ;
#21617=DIRECTION ( 'NONE',  ( 0.000000000000000000, 1.000000000000000000, -0.000000000000000000 ) ) ;
#21630=DIRECTION ( 'NONE',  ( 1.000000000000000000, -0.000000000000000000, -0.000000000000000000 ) ) ;
#21660=CARTESIAN_POINT ( 'NONE',  ( -26.42409385541305511, -15.80920654474410725, 48.99999999999997868 ) ) ;
#21684=ORIENTED_EDGE ( 'NONE', *, *, #19300, .T. ) ;
#21692=DIRECTION ( 'NONE',  ( -0.000000000000000000, -1.000000000000000000, -0.000000000000000000 ) ) ;
#21700=ADVANCED_FACE ( 'NONE', ( #15871 ), #24015, .T. ) ;
#21722=EDGE_CURVE ( 'NONE', #39291, #48597, #4808, .T. ) ;
#21727=VERTEX_POINT ( 'NONE', #1838 ) ;
#21745=EDGE_CURVE ( 'NONE', #45033, #10587, #31571, .T. ) ;
#21765=DIRECTION ( 'NONE',  ( -1.000000000000000000, 0.000000000000000000, 0.000000000000000000 ) ) ;
#21794=AXIS2_PLACEMENT_3D ( 'NONE', #11743, #41286, #41535 ) ;
#21811=EDGE_CURVE ( 'NONE', #112, #39233, #39746, .T. ) ;
#21819=CARTESIAN_POINT ( 'NONE',  ( -8.424093855413071097, -6.859206544744110623, 52.99999999999997868 ) ) ;
#21825=ORIENTED_EDGE ( 'NONE', *, *, #28709, .F. ) ;
#21836=DIRECTION ( 'NONE',  ( 0.000000000000000000, 0.000000000000000000, 1.000000000000000000 ) ) ;
#21837=AXIS2_PLACEMENT_3D ( 'NONE', #48219, #25097, #40120 ) ;
#21861=CARTESIAN_POINT ( 'NONE',  ( -13.92409385541305511, -10.60920654474410618, 78.99999999999998579 ) ) ;
#21876=ADVANCED_FACE ( 'NONE', ( #9723 ), #39992, .T. ) ;
#21881=EDGE_CURVE ( 'NONE', #21727, #10431, #33087, .T. ) ;
#21884=CARTESIAN_POINT ( 'NONE',  ( -17.42409385541305511, -14.80920654474410725, 45.99899999999998101 ) ) ;
#21921=DIRECTION ( 'NONE',  ( -1.000000000000000000, -0.000000000000000000, -0.000000000000000000 ) ) ;
#21940=DIRECTION ( 'NONE',  ( 0.000000000000000000, 0.000000000000000000, -1.000000000000000000 ) ) ;
#21973=CARTESIAN_POINT ( 'NONE',  ( -38.65852941833841783, -27.10920654474410796, 78.99999999999998579 ) ) ;
#21979=CARTESIAN_POINT ( 'NONE',  ( -20.92409385541305511, -10.60920654474410618, 78.99999999999998579 ) ) ;
#22053=VECTOR ( 'NONE', #43246, 1000.000000000000000 ) ;
#22079=DIRECTION ( 'NONE',  ( -0.000000000000000000, -1.000000000000000000, -0.000000000000000000 ) ) ;
#22105=ADVANCED_FACE ( 'NONE', ( #42671 ), #19775, .T. ) ;
#22116=ORIENTED_EDGE ( 'NONE', *, *, #27519, .F. ) ;
#22134=ORIENTED_EDGE ( 'NONE', *, *, #34280, .F. ) ;
#22139=AXIS2_PLACEMENT_3D ( 'NONE', #41258, #33356, #48161 ) ;
#22149=FACE_OUTER_BOUND ( 'NONE', #20180, .T. ) ;
#22182=CARTESIAN_POINT ( 'NONE',  ( -38.65852941833841783, -27.10920654474410796, 76.99999999999998579 ) ) ;
#22185=DIRECTION ( 'NONE',  ( 0.000000000000000000, 1.000000000000000000, -0.000000000000000000 ) ) ;
#22218=EDGE_CURVE ( 'NONE', #20093, #44110, #20476, .T. ) ;
#22271=ORIENTED_EDGE ( 'NONE', *, *, #47313, .F. ) ;
#22287=ORIENTED_EDGE ( 'NONE', *, *, #26839, .T. ) ;
#22293=ORIENTED_EDGE ( 'NONE', *, *, #13746, .T. ) ;
#22303=ORIENTED_EDGE ( 'NONE', *, *, #37086, .T. ) ;
#22310=DIRECTION ( 'NONE',  ( -1.000000000000000000, 0.000000000000000000, 0.000000000000000000 ) ) ;
#22313=ORIENTED_EDGE ( 'NONE', *, *, #8674, .T. ) ;
#22329=LINE ( 'NONE', #47948, #17818 ) ;
#22347=ORIENTED_EDGE ( 'NONE', *, *, #226, .F. ) ;
#22367=AXIS2_PLACEMENT_3D ( 'NONE', #18068, #13645, #44220 ) ;
#22383=LINE ( 'NONE', #18186, #45927 ) ;
#22401=ORIENTED_EDGE ( 'NONE', *, *, #24897, .T. ) ;
#22431=CARTESIAN_POINT ( 'NONE',  ( -6.424093855413058662, -6.359206544744109735, 52.99999999999998579 ) ) ;
#22443=AXIS2_PLACEMENT_3D ( 'NONE', #30033, #42262, #4583 ) ;
#22447=CARTESIAN_POINT ( 'NONE',  ( -16.94712425470457973, -14.65920654474411045, 48.99999999999997868 ) ) ;
#22452=DIRECTION ( 'NONE',  ( 0.000000000000000000, 0.000000000000000000, 1.000000000000000000 ) ) ;
#22489=ORIENTED_EDGE ( 'NONE', *, *, #41877, .T. ) ;
#22497=CARTESIAN_POINT ( 'NONE',  ( -45.92409385541305511, -17.80920654474410370, 69.24999999999998579 ) ) ;
#22506=ORIENTED_EDGE ( 'NONE', *, *, #25100, .T. ) ;
#22508=EDGE_CURVE ( 'NONE', #9150, #14458, #10077, .T. ) ;
#22559=LINE ( 'NONE', #2088, #15288 ) ;
#22564=DIRECTION ( 'NONE',  ( 1.000000000000000000, 0.000000000000000000, 0.000000000000000000 ) ) ;
#22605=EDGE_LOOP ( 'NONE', ( #3197, #42770, #35105, #39748 ) ) ;
#22630=AXIS2_PLACEMENT_3D ( 'NONE', #37999, #16558, #45667 ) ;
#22645=VERTEX_POINT ( 'NONE', #40352 ) ;
#22675=ORIENTED_EDGE ( 'NONE', *, *, #38036, .T. ) ;
#22681=AXIS2_PLACEMENT_3D ( 'NONE', #46327, #32023, #5202 ) ;
#22684=DIRECTION ( 'NONE',  ( -0.000000000000000000, -1.000000000000000000, -0.000000000000000000 ) ) ;
#22718=DIRECTION ( 'NONE',  ( 0.000000000000000000, 0.000000000000000000, 1.000000000000000000 ) ) ;
#22741=ORIENTED_EDGE ( 'NONE', *, *, #39858, .F. ) ;
#22765=VECTOR ( 'NONE', #19118, 1000.000000000000000 ) ;
#22790=CARTESIAN_POINT ( 'NONE',  ( -28.42409385541305511, -6.859206544744110623, 52.99999999999997158 ) ) ;
#22801=AXIS2_PLACEMENT_3D ( 'NONE', #3936, #18942, #41107 ) ;
#22805=DIRECTION ( 'NONE',  ( 1.927470528863119542E-16, 0.000000000000000000, -1.000000000000000000 ) ) ;
#22843=DIRECTION ( 'NONE',  ( 0.000000000000000000, 0.000000000000000000, -1.000000000000000000 ) ) ;
#22868=VECTOR ( 'NONE', #21940, 1000.000000000000000 ) ;
#22887=PLANE ( 'NONE',  #37726 ) ;
#22957=DIRECTION ( 'NONE',  ( 1.000000000000000000, 0.000000000000000000, -5.466375705775733989E-17 ) ) ;
#22967=LINE ( 'NONE', #11142, #38888 ) ;
#22973=ORIENTED_EDGE ( 'NONE', *, *, #24938, .T. ) ;
#22998=DIRECTION ( 'NONE',  ( 0.000000000000000000, -1.000000000000000000, 9.912705577010318647E-16 ) ) ;
#23001=ORIENTED_EDGE ( 'NONE', *, *, #31904, .F. ) ;
#23013=ORIENTED_EDGE ( 'NONE', *, *, #31377, .T. ) ;
#23028=CARTESIAN_POINT ( 'NONE',  ( -50.42409385541304800, -25.10920654474410441, 47.99999999999998579 ) ) ;
#23043=ORIENTED_EDGE ( 'NONE', *, *, #8442, .F. ) ;
#23071=VERTEX_POINT ( 'NONE', #42103 ) ;
#23097=CARTESIAN_POINT ( 'NONE',  ( -17.42409385541305511, -14.80920654474410725, 47.99999999999998579 ) ) ;
#23101=DIRECTION ( 'NONE',  ( -1.000000000000000000, 0.000000000000000000, 0.000000000000000000 ) ) ;
#23155=PLANE ( 'NONE',  #3701 ) ;
#23181=CARTESIAN_POINT ( 'NONE',  ( -30.42409385541305156, -25.10920654474410441, 47.99999999999997868 ) ) ;
#23187=ORIENTED_EDGE ( 'NONE', *, *, #45646, .T. ) ;
#23195=DIRECTION ( 'NONE',  ( 0.000000000000000000, 1.000000000000000000, 0.000000000000000000 ) ) ;
#23232=VECTOR ( 'NONE', #12091, 1000.000000000000000 ) ;
#23234=FACE_OUTER_BOUND ( 'NONE', #6985, .T. ) ;
#23245=PLANE ( 'NONE',  #25122 ) ;
#23258=DIRECTION ( 'NONE',  ( 1.000000000000000000, 0.000000000000000000, 0.000000000000000000 ) ) ;
#23269=DIRECTION ( 'NONE',  ( 1.000000000000000000, 0.000000000000000000, 0.000000000000000000 ) ) ;
#23283=LINE ( 'NONE', #18585, #6356 ) ;
#23342=DIRECTION ( 'NONE',  ( -0.000000000000000000, -1.000000000000000000, -0.000000000000000000 ) ) ;
#23355=LINE ( 'NONE', #38116, #47969 ) ;
#23395=EDGE_CURVE ( 'NONE', #20101, #5342, #38327, .T. ) ;
#23407=ORIENTED_EDGE ( 'NONE', *, *, #42946, .F. ) ;
#23420=FACE_OUTER_BOUND ( 'NONE', #20970, .T. ) ;
#23426=ORIENTED_EDGE ( 'NONE', *, *, #3826, .F. ) ;
#23437=SURFACE_STYLE_FILL_AREA ( #19488 ) ;
#23445=ORIENTED_EDGE ( 'NONE', *, *, #39858, .T. ) ;
#23460=VECTOR ( 'NONE', #33805, 1000.000000000000000 ) ;
#23463=AXIS2_PLACEMENT_3D ( 'NONE', #46631, #36004, #13588 ) ;
#23465=DIRECTION ( 'NONE',  ( 0.000000000000000000, 0.000000000000000000, 1.000000000000000000 ) ) ;
#23477=EDGE_CURVE ( 'NONE', #25709, #30260, #26586, .T. ) ;
#23480=LINE ( 'NONE', #15823, #7791 ) ;
#23487=CARTESIAN_POINT ( 'NONE',  ( -27.42409385541305511, -25.10920654474410441, 45.99999999999998579 ) ) ;
#23504=EDGE_CURVE ( 'NONE', #24008, #20983, #43100, .T. ) ;
#23540=AXIS2_PLACEMENT_3D ( 'NONE', #29118, #24717, #40212 ) ;
#23549=ORIENTED_EDGE ( 'NONE', *, *, #16275, .T. ) ;
#23568=VERTEX_POINT ( 'NONE', #39558 ) ;
#23584=EDGE_CURVE ( 'NONE', #44063, #46918, #5835, .T. ) ;
#23605=CIRCLE ( 'NONE', #8782, 1.250000000000001110 ) ;
#23613=VECTOR ( 'NONE', #13225, 1000.000000000000000 ) ;
#23619=EDGE_LOOP ( 'NONE', ( #26047, #8974, #645, #22116 ) ) ;
#23664=CARTESIAN_POINT ( 'NONE',  ( -13.92409385541305511, -10.10920654474410618, 78.99999999999998579 ) ) ;
#23669=FACE_OUTER_BOUND ( 'NONE', #48586, .T. ) ;
#23697=AXIS2_PLACEMENT_3D ( 'NONE', #11146, #19257, #7219 ) ;
#23700=DIRECTION ( 'NONE',  ( 0.000000000000000000, 0.000000000000000000, 1.000000000000000000 ) ) ;
#23741=CARTESIAN_POINT ( 'NONE',  ( -27.42409385541305511, -15.80920654474410725, 56.99999999999999289 ) ) ;
#23781=DIRECTION ( 'NONE',  ( -0.000000000000000000, 1.000000000000000000, -0.000000000000000000 ) ) ;
#23782=ORIENTED_EDGE ( 'NONE', *, *, #18531, .T. ) ;
#23812=ORIENTED_EDGE ( 'NONE', *, *, #20874, .T. ) ;
#23839=ORIENTED_EDGE ( 'NONE', *, *, #32412, .F. ) ;
#23873=EDGE_CURVE ( 'NONE', #2100, #5464, #43700, .T. ) ;
#23904=CARTESIAN_POINT ( 'NONE',  ( -38.65852941833841783, -25.10920654474410441, 76.99999999999998579 ) ) ;
#23920=DIRECTION ( 'NONE',  ( 0.000000000000000000, 0.000000000000000000, -1.000000000000000000 ) ) ;
#23933=VECTOR ( 'NONE', #28206, 1000.000000000000000 ) ;
#23943=EDGE_CURVE ( 'NONE', #8183, #37009, #25219, .T. ) ;
#23958=DIRECTION ( 'NONE',  ( -0.000000000000000000, -1.000000000000000000, -0.000000000000000000 ) ) ;
#23964=CARTESIAN_POINT ( 'NONE',  ( -20.92409385541305511, -10.60920654474410618, 80.49999999999998579 ) ) ;
#23977=LINE ( 'NONE', #37318, #29812 ) ;
#23982=ORIENTED_EDGE ( 'NONE', *, *, #37134, .T. ) ;
#24008=VERTEX_POINT ( 'NONE', #28903 ) ;
#24010=PLANE ( 'NONE',  #9438 ) ;
#24015=PLANE ( 'NONE',  #18989 ) ;
#24059=CARTESIAN_POINT ( 'NONE',  ( -29.92409385541305156, -6.859206544744110623, 47.99999999999997868 ) ) ;
#24079=ORIENTED_EDGE ( 'NONE', *, *, #41861, .T. ) ;
#24091=ORIENTED_EDGE ( 'NONE', *, *, #19300, .F. ) ;
#24114=FACE_OUTER_BOUND ( 'NONE', #22605, .T. ) ;
#24163=LINE ( 'NONE', #17235, #10792 ) ;
#24170=CIRCLE ( 'NONE', #46968, 1.500000000000001332 ) ;
#24202=CARTESIAN_POINT ( 'NONE',  ( -17.90106345612152694, -14.65920654474411045, 48.99999999999997868 ) ) ;
#24212=ORIENTED_EDGE ( 'NONE', *, *, #10316, .F. ) ;
#24227=ADVANCED_FACE ( 'NONE', ( #47332 ), #35256, .T. ) ;
#24269=DIRECTION ( 'NONE',  ( 0.000000000000000000, 0.000000000000000000, 1.000000000000000000 ) ) ;
#24271=ORIENTED_EDGE ( 'NONE', *, *, #38718, .T. ) ;
#24275=CARTESIAN_POINT ( 'NONE',  ( -27.42409385541305511, -27.10920654474410796, 45.99999999999998579 ) ) ;
#24284=CARTESIAN_POINT ( 'NONE',  ( -27.42409385541305511, -10.60920654474410618, 78.99999999999998579 ) ) ;
#24324=DIRECTION ( 'NONE',  ( -0.000000000000000000, -1.000000000000000000, -0.000000000000000000 ) ) ;
#24337=DIRECTION ( 'NONE',  ( 0.000000000000000000, 1.000000000000000000, -0.000000000000000000 ) ) ;
#24354=DIRECTION ( 'NONE',  ( 0.000000000000000000, 0.000000000000000000, -1.000000000000000000 ) ) ;
#24367=CARTESIAN_POINT ( 'NONE',  ( -30.42409385541305156, -8.109206544744111511, 50.50000000000000000 ) ) ;
#24372=CARTESIAN_POINT ( 'NONE',  ( -8.424093855413071097, -8.109206544744111511, 51.75000000000000000 ) ) ;
#24391=DIRECTION ( 'NONE',  ( 0.000000000000000000, 1.000000000000000000, 0.000000000000000000 ) ) ;
#24467=TOROIDAL_SURFACE ( 'NONE', #3206, 1.500000000000008660, 0.5000000000000000000 ) ;
#24487=ADVANCED_FACE ( 'NONE', ( #37418 ), #45333, .T. ) ;
#24491=VECTOR ( 'NONE', #3921, 1000.000000000000000 ) ;
#24535=ORIENTED_EDGE ( 'NONE', *, *, #13537, .T. ) ;
#24636=ORIENTED_EDGE ( 'NONE', *, *, #6379, .T. ) ;
#24638=DIRECTION ( 'NONE',  ( -0.000000000000000000, -1.000000000000000000, -0.000000000000000000 ) ) ;
#24645=PLANE ( 'NONE',  #38502 ) ;
#24659=ORIENTED_EDGE ( 'NONE', *, *, #2103, .T. ) ;
#24671=VERTEX_POINT ( 'NONE', #21819 ) ;
#24717=DIRECTION ( 'NONE',  ( 1.000000000000000000, -0.000000000000000000, -2.406186529621654511E-16 ) ) ;
#24724=VERTEX_POINT ( 'NONE', #30688 ) ;
#24727=FACE_OUTER_BOUND ( 'NONE', #29185, .T. ) ;
#24816=ORIENTED_EDGE ( 'NONE', *, *, #48610, .T. ) ;
#24839=CIRCLE ( 'NONE', #33447, 1.250000000000001110 ) ;
#24894=CARTESIAN_POINT ( 'NONE',  ( -17.42409385541305511, -14.80920654474410725, 79.00000000000000000 ) ) ;
#24897=EDGE_CURVE ( 'NONE', #30760, #45046, #25228, .T. ) ;
#24900=AXIS2_PLACEMENT_3D ( 'NONE', #21209, #21921, #40162 ) ;
#24903=EDGE_CURVE ( 'NONE', #24008, #6937, #47843, .T. ) ;
#24916=CARTESIAN_POINT ( 'NONE',  ( -50.42409385541304800, -25.10920654474410441, 74.99999999999998579 ) ) ;
#24938=EDGE_CURVE ( 'NONE', #43029, #36353, #16847, .T. ) ;
#24941=CARTESIAN_POINT ( 'NONE',  ( -40.92409385541305511, -15.80920654474410725, 74.99999999999998579 ) ) ;
#24943=CARTESIAN_POINT ( 'NONE',  ( -46.92409385541305511, -17.80920654474410370, 60.24999999999999289 ) ) ;
#24945=EDGE_CURVE ( 'NONE', #4984, #3647, #2215, .T. ) ;
#24954=VERTEX_POINT ( 'NONE', #44435 ) ;
#24957=EDGE_CURVE ( 'NONE', #20146, #37066, #7253, .T. ) ;
#24969=CARTESIAN_POINT ( 'NONE',  ( -17.82409385541305369, -14.80920654474410725, 52.21286476528345588 ) ) ;
#24974=DIRECTION ( 'NONE',  ( 1.000000000000000000, -0.000000000000000000, 0.000000000000000000 ) ) ;
#24982=ORIENTED_EDGE ( 'NONE', *, *, #28242, .F. ) ;
#24985=CARTESIAN_POINT ( 'NONE',  ( -45.92409385541305511, -17.80920654474410370, 71.75000000000000000 ) ) ;
#25050=CYLINDRICAL_SURFACE ( 'NONE', #3226, 2.500000000000000444 ) ;
#25073=VECTOR ( 'NONE', #21229, 1000.000000000000000 ) ;
#25095=EDGE_CURVE ( 'NONE', #45181, #26808, #4760, .T. ) ;
#25097=DIRECTION ( 'NONE',  ( -0.000000000000000000, -1.000000000000000000, -0.000000000000000000 ) ) ;
#25100=EDGE_CURVE ( 'NONE', #115, #38493, #23480, .T. ) ;
#25122=AXIS2_PLACEMENT_3D ( 'NONE', #23487, #38484, #36240 ) ;
#25150=ORIENTED_EDGE ( 'NONE', *, *, #15112, .T. ) ;
#25204=CARTESIAN_POINT ( 'NONE',  ( -48.42409385541304800, -25.10920654474410441, 79.99999999999998579 ) ) ;
#25219=LINE ( 'NONE', #17801, #40695 ) ;
#25228=LINE ( 'NONE', #27941, #15595 ) ;
#25246=EDGE_LOOP ( 'NONE', ( #5811, #42939, #13886, #37060, #27363, #45997 ) ) ;
#25268=ORIENTED_EDGE ( 'NONE', *, *, #8674, .F. ) ;
#25288=VERTEX_POINT ( 'NONE', #43645 ) ;
#25304=AXIS2_PLACEMENT_3D ( 'NONE', #40898, #35, #11113 ) ;
#25308=LINE ( 'NONE', #40319, #17840 ) ;
#25310=EDGE_CURVE ( 'NONE', #27657, #3647, #32067, .T. ) ;
#25312=DIRECTION ( 'NONE',  ( 1.927470528863119542E-16, 0.000000000000000000, -1.000000000000000000 ) ) ;
#25331=DIRECTION ( 'NONE',  ( 1.000000000000000000, -0.000000000000000000, -2.406186529621654511E-16 ) ) ;
#25337=ORIENTED_EDGE ( 'NONE', *, *, #24897, .F. ) ;
#25346=DIRECTION ( 'NONE',  ( -1.000000000000000000, 0.000000000000000000, 0.000000000000000000 ) ) ;
#25373=ADVANCED_FACE ( 'NONE', ( #14284 ), #15021, .T. ) ;
#25391=VERTEX_POINT ( 'NONE', #3721 ) ;
#25419=DIRECTION ( 'NONE',  ( -0.000000000000000000, -1.000000000000000000, 0.000000000000000000 ) ) ;
#25422=CARTESIAN_POINT ( 'NONE',  ( -33.52409385541305653, -2.423472813913224222, 52.29999999999998295 ) ) ;
#25463=VERTEX_POINT ( 'NONE', #36460 ) ;
#25464=CARTESIAN_POINT ( 'NONE',  ( -18.92409385541305511, -14.80920654474410547, 47.99999999999998579 ) ) ;
#25492=ORIENTED_EDGE ( 'NONE', *, *, #41754, .T. ) ;
#25508=LINE ( 'NONE', #14630, #6125 ) ;
#25511=ORIENTED_EDGE ( 'NONE', *, *, #29794, .F. ) ;
#25558=EDGE_CURVE ( 'NONE', #46918, #18891, #46305, .T. ) ;
#25561=AXIS2_PLACEMENT_3D ( 'NONE', #15285, #23195, #38185 ) ;
#25597=ORIENTED_EDGE ( 'NONE', *, *, #44375, .T. ) ;
#25640=EDGE_CURVE ( 'NONE', #10431, #5464, #39637, .T. ) ;
#25649=CARTESIAN_POINT ( 'NONE',  ( -6.424093855413055110, -27.10920654474410796, 45.99999999999998579 ) ) ;
#25668=CIRCLE ( 'NONE', #5263, 0.5000000000000004441 ) ;
#25709=VERTEX_POINT ( 'NONE', #17464 ) ;
#25763=VECTOR ( 'NONE', #24974, 1000.000000000000000 ) ;
#25779=CARTESIAN_POINT ( 'NONE',  ( -26.42409385541305511, -15.80920654474410725, 63.99999999999998579 ) ) ;
#25803=CIRCLE ( 'NONE', #35246, 1.500000000000001332 ) ;
#25912=AXIS2_PLACEMENT_3D ( 'NONE', #30132, #45157, #11398 ) ;
#25928=CIRCLE ( 'NONE', #11768, 2.000000000000001776 ) ;
#25934=CARTESIAN_POINT ( 'NONE',  ( -33.95962776134579286, -8.109206544744111511, 50.50000000000000000 ) ) ;
#25946=DIRECTION ( 'NONE',  ( -1.000000000000000000, 0.000000000000000000, 9.637352644315596475E-17 ) ) ;
#26004=CARTESIAN_POINT ( 'NONE',  ( -33.52409385541305653, -6.359206544744109735, 48.79999999999998295 ) ) ;
#26032=CARTESIAN_POINT ( 'NONE',  ( -27.42409385541305156, -15.80920654474410725, 47.99999999999997868 ) ) ;
#26047=ORIENTED_EDGE ( 'NONE', *, *, #29602, .T. ) ;
#26075=CARTESIAN_POINT ( 'NONE',  ( -28.42409385541305511, -6.859206544744110623, 52.99999999999997158 ) ) ;
#26103=ORIENTED_EDGE ( 'NONE', *, *, #16275, .F. ) ;
#26118=DIRECTION ( 'NONE',  ( 1.000000000000000000, -0.000000000000000000, 2.081668171172170091E-15 ) ) ;
#26119=EDGE_CURVE ( 'NONE', #8183, #11393, #182, .T. ) ;
#26123=DIRECTION ( 'NONE',  ( -0.000000000000000000, -1.000000000000000000, -0.000000000000000000 ) ) ;
#26144=ORIENTED_EDGE ( 'NONE', *, *, #25558, .T. ) ;
#26167=EDGE_CURVE ( 'NONE', #21252, #29761, #23977, .T. ) ;
#26182=EDGE_CURVE ( 'NONE', #1645, #2748, #46381, .T. ) ;
#26187=EDGE_CURVE ( 'NONE', #35729, #17425, #15395, .T. ) ;
#26221=VERTEX_POINT ( 'NONE', #7323 ) ;
#26246=DIRECTION ( 'NONE',  ( 0.000000000000000000, 0.000000000000000000, -1.000000000000000000 ) ) ;
#26269=VERTEX_POINT ( 'NONE', #36000 ) ;
#26280=VECTOR ( 'NONE', #32089, 1000.000000000000000 ) ;
#26294=CARTESIAN_POINT ( 'NONE',  ( -17.42409385541305511, -14.80920654474410725, 52.21286476528345588 ) ) ;
#26390=DIRECTION ( 'NONE',  ( 0.000000000000000000, 0.000000000000000000, -1.000000000000000000 ) ) ;
#26420=CARTESIAN_POINT ( 'NONE',  ( -46.92409385541305511, -15.80920654474410725, 60.24999999999999289 ) ) ;
#26441=ADVANCED_FACE ( 'NONE', ( #9832 ), #36148, .F. ) ;
#26447=DIRECTION ( 'NONE',  ( 0.000000000000000000, 0.000000000000000000, 1.000000000000000000 ) ) ;
#26458=EDGE_CURVE ( 'NONE', #27657, #33767, #47259, .T. ) ;
#26488=DIRECTION ( 'NONE',  ( 1.000000000000000000, -0.000000000000000000, -2.406186529621654511E-16 ) ) ;
#26508=ORIENTED_EDGE ( 'NONE', *, *, #4205, .F. ) ;
#26537=ORIENTED_EDGE ( 'NONE', *, *, #19217, .F. ) ;
#26557=EDGE_LOOP ( 'NONE', ( #3944, #24212, #13534, #29439, #4818 ) ) ;
#26567=AXIS2_PLACEMENT_3D ( 'NONE', #20994, #35523, #46625 ) ;
#26586=CIRCLE ( 'NONE', #33615, 1.999999999999994893 ) ;
#26597=EDGE_CURVE ( 'NONE', #24724, #1836, #39127, .T. ) ;
#26610=VERTEX_POINT ( 'NONE', #46770 ) ;
#26644=CARTESIAN_POINT ( 'NONE',  ( -27.42409385541305511, -25.10920654474410441, 78.99999999999998579 ) ) ;
#26648=DIRECTION ( 'NONE',  ( -0.000000000000000000, -1.000000000000000000, 0.000000000000000000 ) ) ;
#26662=EDGE_CURVE ( 'NONE', #17465, #1836, #21402, .T. ) ;
#26715=DIRECTION ( 'NONE',  ( -0.000000000000000000, -1.000000000000000000, -0.000000000000000000 ) ) ;
#26752=FACE_OUTER_BOUND ( 'NONE', #34584, .T. ) ;
#26753=CARTESIAN_POINT ( 'NONE',  ( -40.64308517176574753, -27.10920654474410796, 77.24806946917840378 ) ) ;
#26766=TOROIDAL_SURFACE ( 'NONE', #40907, 1.499999999999998224, 0.5000000000000000000 ) ;
#26779=VECTOR ( 'NONE', #5356, 1000.000000000000000 ) ;
#26808=VERTEX_POINT ( 'NONE', #34582 ) ;
#26839=EDGE_CURVE ( 'NONE', #41762, #11480, #48702, .T. ) ;
#26840=AXIS2_PLACEMENT_3D ( 'NONE', #16599, #34831, #34585 ) ;
#26865=AXIS2_PLACEMENT_3D ( 'NONE', #8253, #23269, #3823 ) ;
#26890=FACE_OUTER_BOUND ( 'NONE', #41571, .T. ) ;
#26899=DIRECTION ( 'NONE',  ( 0.000000000000000000, 0.000000000000000000, 1.000000000000000000 ) ) ;
#26905=VECTOR ( 'NONE', #20113, 1000.000000000000000 ) ;
#26927=DIRECTION ( 'NONE',  ( 1.000000000000000000, 0.000000000000000000, 0.000000000000000000 ) ) ;
#26936=CARTESIAN_POINT ( 'NONE',  ( -26.42409385541305511, -6.859206544744110623, 47.99999999999997868 ) ) ;
#26964=CARTESIAN_POINT ( 'NONE',  ( -17.79490377976783932, -14.65920654474411045, 48.99999999999997868 ) ) ;
#26974=CARTESIAN_POINT ( 'NONE',  ( -6.424093855413055110, -25.10920654474410441, 79.99999999999998579 ) ) ;
#26983=FACE_OUTER_BOUND ( 'NONE', #37686, .T. ) ;
#26987=EDGE_LOOP ( 'NONE', ( #37511, #35038, #7198, #42306 ) ) ;
#26996=ADVANCED_FACE ( 'NONE', ( #43206 ), #24010, .T. ) ;
#27013=FACE_OUTER_BOUND ( 'NONE', #27594, .T. ) ;
#27063=ORIENTED_EDGE ( 'NONE', *, *, #10574, .T. ) ;
#27075=DIRECTION ( 'NONE',  ( 0.000000000000000000, 0.000000000000000000, 1.000000000000000000 ) ) ;
#27083=VECTOR ( 'NONE', #40846, 1000.000000000000000 ) ;
#27097=EDGE_CURVE ( 'NONE', #17527, #33284, #33290, .T. ) ;
#27102=CYLINDRICAL_SURFACE ( 'NONE', #6128, 0.5000000000000004441 ) ;
#27120=AXIS2_PLACEMENT_3D ( 'NONE', #8900, #42868, #23920 ) ;
#27121=CARTESIAN_POINT ( 'NONE',  ( -35.32409385541306079, -2.423472813913224222, 48.79999999999998295 ) ) ;
#27160=VECTOR ( 'NONE', #47097, 1000.000000000000000 ) ;
#27186=CARTESIAN_POINT ( 'NONE',  ( -26.42409385541305511, -8.109206544744111511, 50.50000000000000000 ) ) ;
#27187=CARTESIAN_POINT ( 'NONE',  ( -48.42409385541304800, -27.10920654474410796, 79.99999999999998579 ) ) ;
#27208=CARTESIAN_POINT ( 'NONE',  ( -27.42409385541305511, -6.359206544744109735, 63.99999999999998579 ) ) ;
#27246=DIRECTION ( 'NONE',  ( 0.000000000000000000, 1.000000000000000000, -0.000000000000000000 ) ) ;
#27257=AXIS2_PLACEMENT_3D ( 'NONE', #24059, #2123, #13180 ) ;
#27261=DIRECTION ( 'NONE',  ( 0.000000000000000000, 1.000000000000000000, -0.000000000000000000 ) ) ;
#27267=ADVANCED_FACE ( 'NONE', ( #37479 ), #28305, .T. ) ;
#27286=DIRECTION ( 'NONE',  ( 0.000000000000000000, 0.000000000000000000, -1.000000000000000000 ) ) ;
#27292=AXIS2_PLACEMENT_3D ( 'NONE', #9947, #17318, #32367 ) ;
#27295=ORIENTED_EDGE ( 'NONE', *, *, #37134, .F. ) ;
#27320=VECTOR ( 'NONE', #37146, 1000.000000000000000 ) ;
#27363=ORIENTED_EDGE ( 'NONE', *, *, #21286, .T. ) ;
#27365=LINE ( 'NONE', #16983, #29004 ) ;
#27397=VECTOR ( 'NONE', #26488, 1000.000000000000000 ) ;
#27451=CARTESIAN_POINT ( 'NONE',  ( -17.82409385541305369, -14.80920654474410725, 47.99999999999998579 ) ) ;
#27465=EDGE_CURVE ( 'NONE', #44063, #29613, #2252, .T. ) ;
#27495=VECTOR ( 'NONE', #48329, 1000.000000000000000 ) ;
#27500=AXIS2_PLACEMENT_3D ( 'NONE', #38860, #42320, #1181 ) ;
#27505=VECTOR ( 'NONE', #35689, 1000.000000000000000 ) ;
#27508=ADVANCED_FACE ( 'NONE', ( #10384 ), #26766, .T. ) ;
#27519=EDGE_CURVE ( 'NONE', #45418, #26221, #31461, .T. ) ;
#27562=CIRCLE ( 'NONE', #29138, 1.250000000000001110 ) ;
#27586=CARTESIAN_POINT ( 'NONE',  ( -20.92409385541305511, -10.10920654474410618, 78.99999999999998579 ) ) ;
#27590=DIRECTION ( 'NONE',  ( 2.081668171172170091E-15, 0.000000000000000000, -1.000000000000000000 ) ) ;
#27594=EDGE_LOOP ( 'NONE', ( #30785, #5482, #2465, #992 ) ) ;
#27598=CARTESIAN_POINT ( 'NONE',  ( -33.52409385541305653, -6.359206544744109735, 52.29999999999998295 ) ) ;
#27609=( NAMED_UNIT ( * ) PLANE_ANGLE_UNIT ( ) SI_UNIT ( $, .RADIAN. ) );
#27621=CIRCLE ( 'NONE', #40974, 0.5000000000000004441 ) ;
#27630=ADVANCED_FACE ( 'NONE', ( #30800 ), #45818, .T. ) ;
#27646=CARTESIAN_POINT ( 'NONE',  ( -7.424093855413048892, -25.10920654474410441, 63.99999999999998579 ) ) ;
#27647=DIRECTION ( 'NONE',  ( -0.000000000000000000, -1.000000000000000000, -0.000000000000000000 ) ) ;
#27657=VERTEX_POINT ( 'NONE', #46549 ) ;
#27658=LINE ( 'NONE', #1300, #15016 ) ;
#27668=CIRCLE ( 'NONE', #48114, 0.3999999999999975797 ) ;
#27677=DIRECTION ( 'NONE',  ( -0.000000000000000000, -1.000000000000000000, -0.000000000000000000 ) ) ;
#27692=ORIENTED_EDGE ( 'NONE', *, *, #26597, .F. ) ;
#27699=CARTESIAN_POINT ( 'NONE',  ( -6.424093855413055110, -25.10920654474410441, 45.99999999999998579 ) ) ;
#27754=DIRECTION ( 'NONE',  ( -0.000000000000000000, -1.000000000000000000, -0.000000000000000000 ) ) ;
#27775=FACE_OUTER_BOUND ( 'NONE', #45810, .T. ) ;
#27788=VERTEX_POINT ( 'NONE', #29273 ) ;
#27806=DIRECTION ( 'NONE',  ( 0.000000000000000000, 1.000000000000000000, -0.000000000000000000 ) ) ;
#27823=ORIENTED_EDGE ( 'NONE', *, *, #27465, .F. ) ;
#27834=ORIENTED_EDGE ( 'NONE', *, *, #38866, .T. ) ;
#27864=VERTEX_POINT ( 'NONE', #10323 ) ;
#27867=EDGE_LOOP ( 'NONE', ( #15915, #41013, #42108, #17863 ) ) ;
#27876=CARTESIAN_POINT ( 'NONE',  ( -26.42409385541305511, -15.80920654474410725, 48.99999999999997868 ) ) ;
#27885=DIRECTION ( 'NONE',  ( 0.000000000000000000, 0.000000000000000000, 1.000000000000000000 ) ) ;
#27896=FACE_OUTER_BOUND ( 'NONE', #13385, .T. ) ;
#27899=CARTESIAN_POINT ( 'NONE',  ( -4.424093855413053333, -27.10920654474410796, 63.99999999999998579 ) ) ;
#27906=DIRECTION ( 'NONE',  ( -0.000000000000000000, -1.000000000000000000, 0.000000000000000000 ) ) ;
#27941=CARTESIAN_POINT ( 'NONE',  ( -30.42409385541305156, -6.359206544744109735, 52.99999999999997158 ) ) ;
#27977=LINE ( 'NONE', #31683, #34722 ) ;
#27985=CARTESIAN_POINT ( 'NONE',  ( -41.15852941833841783, -27.10920654474410796, 56.99999999999997868 ) ) ;
#27994=VERTEX_POINT ( 'NONE', #9297 ) ;
#27998=LINE ( 'NONE', #20134, #36023 ) ;
#28004=ORIENTED_EDGE ( 'NONE', *, *, #18650, .F. ) ;
#28019=DIRECTION ( 'NONE',  ( 0.000000000000000000, 1.000000000000000000, -0.000000000000000000 ) ) ;
#28048=ORIENTED_EDGE ( 'NONE', *, *, #4235, .F. ) ;
#28075=ORIENTED_EDGE ( 'NONE', *, *, #5890, .F. ) ;
#28078=ADVANCED_FACE ( 'NONE', ( #16168 ), #8330, .T. ) ;
#28117=EDGE_LOOP ( 'NONE', ( #10064, #48019, #4560, #13260, #35150, #18559, #22506, #30883, #38637, #24816 ) ) ;
#28157=CARTESIAN_POINT ( 'NONE',  ( -19.92409385541305511, -14.80920654474410725, 79.00000000000000000 ) ) ;
#28166=CARTESIAN_POINT ( 'NONE',  ( -50.42409385541304800, -25.10920654474410441, 47.99999999999998579 ) ) ;
#28203=VECTOR ( 'NONE', #40320, 1000.000000000000000 ) ;
#28206=DIRECTION ( 'NONE',  ( 1.000000000000000000, 0.000000000000000000, -8.260587980841940012E-17 ) ) ;
#28216=DIRECTION ( 'NONE',  ( -1.000000000000000000, 0.000000000000000000, 0.000000000000000000 ) ) ;
#28218=VERTEX_POINT ( 'NONE', #31937 ) ;
#28230=AXIS2_PLACEMENT_3D ( 'NONE', #37181, #43891, #6926 ) ;
#28236=CARTESIAN_POINT ( 'NONE',  ( -6.424093855413058662, -6.359206544744109735, 52.99999999999998579 ) ) ;
#28241=CARTESIAN_POINT ( 'NONE',  ( -9.424093855413055110, -25.10920654474410441, 56.99999999999997868 ) ) ;
#28242=EDGE_CURVE ( 'NONE', #26610, #39233, #27562, .T. ) ;
#28246=CARTESIAN_POINT ( 'NONE',  ( -13.92409385541305511, -25.10920654474410441, 80.49999999999998579 ) ) ;
#28288=DIRECTION ( 'NONE',  ( -0.000000000000000000, -1.000000000000000000, 0.000000000000000000 ) ) ;
#28305=TOROIDAL_SURFACE ( 'NONE', #25912, 1.500000000000008660, 0.5000000000000000000 ) ;
#28311=EDGE_LOOP ( 'NONE', ( #25337, #10572, #23407, #33039, #23839, #45914, #39865, #3542 ) ) ;
#28326=ORIENTED_EDGE ( 'NONE', *, *, #30506, .F. ) ;
#28376=DIRECTION ( 'NONE',  ( 0.000000000000000000, 0.000000000000000000, -1.000000000000000000 ) ) ;
#28396=ORIENTED_EDGE ( 'NONE', *, *, #32444, .F. ) ;
#28398=AXIS2_PLACEMENT_3D ( 'NONE', #5881, #13487, #24354 ) ;
#28466=DIRECTION ( 'NONE',  ( 2.181982678098338148E-16, 0.000000000000000000, -1.000000000000000000 ) ) ;
#28469=CARTESIAN_POINT ( 'NONE',  ( -17.02409385541305653, -14.80920654474410725, 52.21286476528345588 ) ) ;
#28521=EDGE_CURVE ( 'NONE', #30462, #4687, #14510, .T. ) ;
#28555=EDGE_LOOP ( 'NONE', ( #47956, #46256, #8945, #22741 ) ) ;
#28578=CARTESIAN_POINT ( 'NONE',  ( -26.42409385541305511, -6.859206544744110623, 63.99999999999998579 ) ) ;
#28593=LINE ( 'NONE', #41357, #40985 ) ;
#28635=CARTESIAN_POINT ( 'NONE',  ( -6.424093855413058662, -6.859206544744110623, 54.49999999999999289 ) ) ;
#28640=CARTESIAN_POINT ( 'NONE',  ( -33.52409385541305653, -25.10920654474410441, 48.79999999999998295 ) ) ;
#28641=VERTEX_POINT ( 'NONE', #37680 ) ;
#28665=CIRCLE ( 'NONE', #22367, 2.000000000000001776 ) ;
#28671=CIRCLE ( 'NONE', #37284, 0.5000000000000004441 ) ;
#28697=ORIENTED_EDGE ( 'NONE', *, *, #26662, .F. ) ;
#28709=EDGE_CURVE ( 'NONE', #3895, #2100, #15769, .T. ) ;
#28718=LINE ( 'NONE', #10496, #33921 ) ;
#28719=DIRECTION ( 'NONE',  ( 0.000000000000000000, 0.000000000000000000, 1.000000000000000000 ) ) ;
#28730=CIRCLE ( 'NONE', #14518, 0.3999999999999975797 ) ;
#28764=CYLINDRICAL_SURFACE ( 'NONE', #4409, 1.250000000000001110 ) ;
#28767=AXIS2_PLACEMENT_3D ( 'NONE', #47767, #2941, #47539 ) ;
#28785=CYLINDRICAL_SURFACE ( 'NONE', #21837, 1.999999999999994893 ) ;
#28804=ORIENTED_EDGE ( 'NONE', *, *, #34501, .T. ) ;
#28816=FACE_OUTER_BOUND ( 'NONE', #37474, .T. ) ;
#28826=EDGE_CURVE ( 'NONE', #30092, #21727, #36163, .T. ) ;
#28836=ORIENTED_EDGE ( 'NONE', *, *, #42975, .T. ) ;
#28891=ADVANCED_FACE ( 'NONE', ( #6870 ), #6389, .F. ) ;
#28896=LINE ( 'NONE', #39988, #45414 ) ;
#28903=CARTESIAN_POINT ( 'NONE',  ( -26.42409385541305511, -6.859206544744110623, 52.99999999999997158 ) ) ;
#28911=EDGE_LOOP ( 'NONE', ( #41464, #3623, #39175, #4010, #46922 ) ) ;
#28930=AXIS2_PLACEMENT_3D ( 'NONE', #2371, #6314, #28719 ) ;
#28940=DIRECTION ( 'NONE',  ( 0.000000000000000000, 0.000000000000000000, 1.000000000000000000 ) ) ;
#28963=VERTEX_POINT ( 'NONE', #41090 ) ;
#28980=ORIENTED_EDGE ( 'NONE', *, *, #10175, .F. ) ;
#28993=CARTESIAN_POINT ( 'NONE',  ( -35.32409385541306079, -8.109206544744111511, 50.49999999999998579 ) ) ;
#29004=VECTOR ( 'NONE', #36190, 1000.000000000000000 ) ;
#29031=AXIS2_PLACEMENT_3D ( 'NONE', #29301, #44568, #33698 ) ;
#29042=EDGE_CURVE ( 'NONE', #36353, #8191, #41330, .T. ) ;
#29057=CARTESIAN_POINT ( 'NONE',  ( -27.42409385541305511, -25.10920654474410441, 45.99999999999998579 ) ) ;
#29109=DIRECTION ( 'NONE',  ( 0.000000000000000000, -1.000000000000000000, 0.000000000000000000 ) ) ;
#29118=CARTESIAN_POINT ( 'NONE',  ( -33.95962776134579286, -8.109206544744111511, 50.50000000000000000 ) ) ;
#29119=DIRECTION ( 'NONE',  ( 0.000000000000000000, 0.000000000000000000, 1.000000000000000000 ) ) ;
#29138=AXIS2_PLACEMENT_3D ( 'NONE', #8048, #33607, #26246 ) ;
#29165=LINE ( 'NONE', #32140, #21214 ) ;
#29171=ORIENTED_EDGE ( 'NONE', *, *, #36980, .F. ) ;
#29184=AXIS2_PLACEMENT_3D ( 'NONE', #36328, #9997, #32642 ) ;
#29185=EDGE_LOOP ( 'NONE', ( #1796, #41913, #7095, #32656 ) ) ;
#29223=LINE ( 'NONE', #44260, #730 ) ;
#29245=ADVANCED_FACE ( 'NONE', ( #10024 ), #25050, .F. ) ;
#29246=CIRCLE ( 'NONE', #2490, 1.250000000000001110 ) ;
#29273=CARTESIAN_POINT ( 'NONE',  ( -43.14308517176575464, -25.10920654474410441, 57.24806946917839667 ) ) ;
#29301=CARTESIAN_POINT ( 'NONE',  ( 0.000000000000000000, 0.000000000000000000, 0.000000000000000000 ) ) ;
#29307=LINE ( 'NONE', #10834, #20183 ) ;
#29324=DIRECTION ( 'NONE',  ( 0.000000000000000000, 0.000000000000000000, 1.000000000000000000 ) ) ;
#29346=ORIENTED_EDGE ( 'NONE', *, *, #26458, .T. ) ;
#29374=CYLINDRICAL_SURFACE ( 'NONE', #40564, 1.250000000000007994 ) ;
#29408=DIRECTION ( 'NONE',  ( -1.000000000000000000, -0.000000000000000000, 8.260587980841940012E-17 ) ) ;
#29439=ORIENTED_EDGE ( 'NONE', *, *, #500, .F. ) ;
#29462=CARTESIAN_POINT ( 'NONE',  ( -4.424093855413056886, -25.10920654474410441, 47.99999999999998579 ) ) ;
#29469=DIRECTION ( 'NONE',  ( -9.637352644315596475E-17, 0.000000000000000000, -1.000000000000000000 ) ) ;
#29471=PRODUCT_DEFINITION ( 'UNKNOWN', '', #31393, #35146 ) ;
#29516=DIRECTION ( 'NONE',  ( -0.000000000000000000, -0.000000000000000000, 1.000000000000000000 ) ) ;
#29526=CYLINDRICAL_SURFACE ( 'NONE', #22443, 1.000000000000000888 ) ;
#29544=ORIENTED_EDGE ( 'NONE', *, *, #43249, .F. ) ;
#29548=CARTESIAN_POINT ( 'NONE',  ( -17.42409385541305511, -14.80920654474410725, 47.99999999999998579 ) ) ;
#29602=EDGE_CURVE ( 'NONE', #45418, #28218, #37758, .T. ) ;
#29613=VERTEX_POINT ( 'NONE', #29906 ) ;
#29623=CARTESIAN_POINT ( 'NONE',  ( -17.42409385541305511, -14.80920654474410725, 81.99999999999998579 ) ) ;
#29630=EDGE_CURVE ( 'NONE', #30602, #12986, #29650, .T. ) ;
#29644=CIRCLE ( 'NONE', #8421, 2.500000000000000444 ) ;
#29650=LINE ( 'NONE', #44442, #32385 ) ;
#29665=DIRECTION ( 'NONE',  ( 0.000000000000000000, 0.000000000000000000, -1.000000000000000000 ) ) ;
#29680=CIRCLE ( 'NONE', #2158, 1.000000000000000888 ) ;
#29691=CARTESIAN_POINT ( 'NONE',  ( -4.424093855413049781, -6.359206544744109735, 52.99999999999998579 ) ) ;
#29699=DIRECTION ( 'NONE',  ( 0.000000000000000000, 0.000000000000000000, 1.000000000000000000 ) ) ;
#29705=LINE ( 'NONE', #29462, #33699 ) ;
#29717=ORIENTED_EDGE ( 'NONE', *, *, #23477, .T. ) ;
#29728=CIRCLE ( 'NONE', #41493, 2.000000000000001776 ) ;
#29755=EDGE_LOOP ( 'NONE', ( #15184, #40021, #36951, #551, #11101 ) ) ;
#29761=VERTEX_POINT ( 'NONE', #1552 ) ;
#29765=DIRECTION ( 'NONE',  ( 0.000000000000000000, 0.000000000000000000, 1.000000000000000000 ) ) ;
#29779=ORIENTED_EDGE ( 'NONE', *, *, #13351, .T. ) ;
#29789=CIRCLE ( 'NONE', #38412, 2.000000000000008882 ) ;
#29794=EDGE_CURVE ( 'NONE', #39884, #38652, #27658, .T. ) ;
#29800=EDGE_CURVE ( 'NONE', #25288, #22645, #46130, .T. ) ;
#29803=DIRECTION ( 'NONE',  ( 0.000000000000000000, 0.000000000000000000, 1.000000000000000000 ) ) ;
#29812=VECTOR ( 'NONE', #41276, 1000.000000000000000 ) ;
#29830=DIRECTION ( 'NONE',  ( 0.000000000000000000, 1.000000000000000000, -0.000000000000000000 ) ) ;
#29841=ORIENTED_EDGE ( 'NONE', *, *, #21333, .F. ) ;
#29842=CARTESIAN_POINT ( 'NONE',  ( -4.424093855413053333, -25.10920654474410441, 63.99999999999998579 ) ) ;
#29906=CARTESIAN_POINT ( 'NONE',  ( -8.424093855413063991, -25.10920654474410441, 48.99999999999997868 ) ) ;
#29939=DIRECTION ( 'NONE',  ( -1.000000000000000000, 0.000000000000000000, 9.637352644315596475E-17 ) ) ;
#29998=CYLINDRICAL_SURFACE ( 'NONE', #43942, 0.3999999999999975797 ) ;
#30018=AXIS2_PLACEMENT_3D ( 'NONE', #46367, #45886, #11909 ) ;
#30033=CARTESIAN_POINT ( 'NONE',  ( -15.92409385541305333, -14.80920654474410547, 52.21286476528345588 ) ) ;
#30034=ADVANCED_FACE ( 'NONE', ( #11319 ), #40861, .F. ) ;
#30092=VERTEX_POINT ( 'NONE', #36656 ) ;
#30132=CARTESIAN_POINT ( 'NONE',  ( -6.424093855413058662, -6.859206544744110623, 52.99999999999998579 ) ) ;
#30142=CARTESIAN_POINT ( 'NONE',  ( -27.42409385541305156, -14.65920654474411045, 48.99999999999997868 ) ) ;
#30150=CARTESIAN_POINT ( 'NONE',  ( -50.42409385541304800, -15.80920654474410725, 74.99999999999998579 ) ) ;
#30165=DIRECTION ( 'NONE',  ( 0.000000000000000000, 0.000000000000000000, 1.000000000000000000 ) ) ;
#30216=ORIENTED_EDGE ( 'NONE', *, *, #43381, .T. ) ;
#30260=VERTEX_POINT ( 'NONE', #35883 ) ;
#30268=CARTESIAN_POINT ( 'NONE',  ( -20.92409385541305511, -25.10920654474410441, 78.99999999999998579 ) ) ;
#30278=ORIENTED_EDGE ( 'NONE', *, *, #48546, .T. ) ;
#30329=DIRECTION ( 'NONE',  ( -0.000000000000000000, -1.000000000000000000, -0.000000000000000000 ) ) ;
#30348=DIRECTION ( 'NONE',  ( -9.637352644315596475E-17, 0.000000000000000000, -1.000000000000000000 ) ) ;
#30351=FACE_OUTER_BOUND ( 'NONE', #19513, .T. ) ;
#30381=ORIENTED_EDGE ( 'NONE', *, *, #12122, .T. ) ;
#30432=DIRECTION ( 'NONE',  ( 0.000000000000000000, 0.000000000000000000, 1.000000000000000000 ) ) ;
#30435=ORIENTED_EDGE ( 'NONE', *, *, #23584, .F. ) ;
#30439=EDGE_LOOP ( 'NONE', ( #4768, #35357, #28836, #6639 ) ) ;
#30462=VERTEX_POINT ( 'NONE', #42708 ) ;
#30500=CARTESIAN_POINT ( 'NONE',  ( -8.424093855413063991, -15.80920654474410725, 48.99999999999997868 ) ) ;
#30506=EDGE_CURVE ( 'NONE', #48597, #17465, #6439, .T. ) ;
#30509=ORIENTED_EDGE ( 'NONE', *, *, #42892, .F. ) ;
#30526=PLANE ( 'NONE',  #32260 ) ;
#30575=VECTOR ( 'NONE', #19847, 1000.000000000000000 ) ;
#30602=VERTEX_POINT ( 'NONE', #28157 ) ;
#30661=DIRECTION ( 'NONE',  ( -0.000000000000000000, -1.000000000000000000, -0.000000000000000000 ) ) ;
#30662=CARTESIAN_POINT ( 'NONE',  ( -30.42409385541305156, -8.109206544744111511, 49.25000000000000000 ) ) ;
#30673=ORIENTED_EDGE ( 'NONE', *, *, #4312, .T. ) ;
#30688=CARTESIAN_POINT ( 'NONE',  ( -6.424093855413055110, -25.10920654474410441, 81.99999999999998579 ) ) ;
#30697=EDGE_CURVE ( 'NONE', #42591, #6937, #35538, .T. ) ;
#30706=EDGE_CURVE ( 'NONE', #18406, #17425, #10379, .T. ) ;
#30757=EDGE_CURVE ( 'NONE', #41525, #26808, #15787, .T. ) ;
#30760=VERTEX_POINT ( 'NONE', #16027 ) ;
#30785=ORIENTED_EDGE ( 'NONE', *, *, #32969, .F. ) ;
#30789=CARTESIAN_POINT ( 'NONE',  ( -29.92409385541305156, -6.359206544744109735, 47.99999999999997868 ) ) ;
#30795=CARTESIAN_POINT ( 'NONE',  ( -6.424093855413055110, -25.10920654474410441, 81.99999999999998579 ) ) ;
#30800=FACE_OUTER_BOUND ( 'NONE', #45084, .T. ) ;
#30803=AXIS2_PLACEMENT_3D ( 'NONE', #24894, #9877, #5709 ) ;
#30813=LINE ( 'NONE', #34473, #41832 ) ;
#30832=DIRECTION ( 'NONE',  ( 1.000000000000000000, 0.000000000000000000, 0.000000000000000000 ) ) ;
#30852=PLANE ( 'NONE',  #10697 ) ;
#30883=ORIENTED_EDGE ( 'NONE', *, *, #9495, .F. ) ;
#30894=DIRECTION ( 'NONE',  ( 0.000000000000000000, 1.000000000000000000, -0.000000000000000000 ) ) ;
#30918=DIRECTION ( 'NONE',  ( 0.000000000000000000, 1.000000000000000000, -0.000000000000000000 ) ) ;
#30943=DIRECTION ( 'NONE',  ( -0.000000000000000000, -1.000000000000000000, -0.000000000000000000 ) ) ;
#30947=ORIENTED_EDGE ( 'NONE', *, *, #13703, .T. ) ;
#31004=PLANE ( 'NONE',  #47543 ) ;
#31027=VECTOR ( 'NONE', #8888, 1000.000000000000000 ) ;
#31036=ORIENTED_EDGE ( 'NONE', *, *, #45240, .T. ) ;
#31051=ORIENTED_EDGE ( 'NONE', *, *, #43585, .F. ) ;
#31064=VECTOR ( 'NONE', #25312, 1000.000000000000000 ) ;
#31084=ORIENTED_EDGE ( 'NONE', *, *, #13017, .T. ) ;
#31094=CARTESIAN_POINT ( 'NONE',  ( -13.92409385541305511, -10.10920654474410618, 80.49999999999998579 ) ) ;
#31120=VERTEX_POINT ( 'NONE', #20164 ) ;
#31149=ORIENTED_EDGE ( 'NONE', *, *, #29602, .F. ) ;
#31166=VERTEX_POINT ( 'NONE', #43799 ) ;
#31168=DIRECTION ( 'NONE',  ( 1.000000000000000000, 0.000000000000000000, -8.260587980841940012E-17 ) ) ;
#31176=ORIENTED_EDGE ( 'NONE', *, *, #23504, .F. ) ;
#31190=CARTESIAN_POINT ( 'NONE',  ( -17.42409385541305511, -14.80920654474410725, 52.21286476528345588 ) ) ;
#31206=CARTESIAN_POINT ( 'NONE',  ( -50.42409385541304800, -27.10920654474410796, 63.99999999999998579 ) ) ;
#31278=VERTEX_POINT ( 'NONE', #10774 ) ;
#31282=CARTESIAN_POINT ( 'NONE',  ( -40.64308517176574753, -25.10920654474410441, 77.24806946917840378 ) ) ;
#31290=CARTESIAN_POINT ( 'NONE',  ( -28.42409385541305511, -6.359206544744109735, 45.99999999999998579 ) ) ;
#31303=DIRECTION ( 'NONE',  ( -0.000000000000000000, -1.000000000000000000, -0.000000000000000000 ) ) ;
#31308=ADVANCED_FACE ( 'NONE', ( #6840 ), #11025, .T. ) ;
#31325=EDGE_CURVE ( 'NONE', #35729, #5074, #40809, .T. ) ;
#31327=VECTOR ( 'NONE', #12925, 1000.000000000000000 ) ;
#31340=CARTESIAN_POINT ( 'NONE',  ( -17.92409385541305511, -14.80920654474410725, 52.21286476528345588 ) ) ;
#31342=DIRECTION ( 'NONE',  ( -1.000000000000000000, 0.000000000000000000, 3.652049423109068320E-16 ) ) ;
#31347=LINE ( 'NONE', #23741, #11624 ) ;
#31375=AXIS2_PLACEMENT_3D ( 'NONE', #42742, #9010, #20328 ) ;
#31377=EDGE_CURVE ( 'NONE', #12986, #27864, #38585, .T. ) ;
#31380=DIRECTION ( 'NONE',  ( 0.1240347345892083841, 0.000000000000000000, 0.9922778767136676281 ) ) ;
#31393=PRODUCT_DEFINITION_FORMATION_WITH_SPECIFIED_SOURCE ( 'ANY', '', #8746, .NOT_KNOWN. ) ;
#31394=DIRECTION ( 'NONE',  ( 0.000000000000000000, 0.000000000000000000, -1.000000000000000000 ) ) ;
#31395=ORIENTED_EDGE ( 'NONE', *, *, #14146, .F. ) ;
#31428=CARTESIAN_POINT ( 'NONE',  ( -7.424093855413048892, -25.10920654474410441, 77.00000000000000000 ) ) ;
#31444=DIRECTION ( 'NONE',  ( -0.000000000000000000, -1.000000000000000000, -0.000000000000000000 ) ) ;
#31448=CARTESIAN_POINT ( 'NONE',  ( -35.32409385541306079, -2.423472813913224222, 52.29999999999998295 ) ) ;
#31453=ORIENTED_EDGE ( 'NONE', *, *, #46174, .T. ) ;
#31456=ORIENTED_EDGE ( 'NONE', *, *, #48142, .T. ) ;
#31461=CIRCLE ( 'NONE', #14916, 1.999999999999994893 ) ;
#31513=DIRECTION ( 'NONE',  ( 0.000000000000000000, 0.000000000000000000, -1.000000000000000000 ) ) ;
#31526=VERTEX_POINT ( 'NONE', #40036 ) ;
#31539=LINE ( 'NONE', #31290, #13868 ) ;
#31544=CARTESIAN_POINT ( 'NONE',  ( -27.42409385541305156, -15.80920654474410725, 74.99999999999998579 ) ) ;
#31555=EDGE_LOOP ( 'NONE', ( #21684, #18809, #47675, #30509, #39450 ) ) ;
#31558=TOROIDAL_SURFACE ( 'NONE', #19792, 1.500000000000000000, 0.5000000000000000000 ) ;
#31560=ORIENTED_EDGE ( 'NONE', *, *, #8269, .T. ) ;
#31571=CIRCLE ( 'NONE', #26840, 2.000000000000008882 ) ;
#31579=FACE_OUTER_BOUND ( 'NONE', #9447, .T. ) ;
#31588=FACE_OUTER_BOUND ( 'NONE', #5358, .T. ) ;
#31615=AXIS2_PLACEMENT_3D ( 'NONE', #11379, #41413, #22718 ) ;
#31623=ORIENTED_EDGE ( 'NONE', *, *, #4235, .T. ) ;
#31630=EDGE_CURVE ( 'NONE', #5074, #17144, #16399, .T. ) ;
#31660=LINE ( 'NONE', #24275, #32178 ) ;
#31667=CARTESIAN_POINT ( 'NONE',  ( -28.42409385541305511, -6.359206544744109735, 52.99999999999997158 ) ) ;
#31683=CARTESIAN_POINT ( 'NONE',  ( -33.95962776134579286, -8.109206544744111511, 49.25000000000000000 ) ) ;
#31691=CIRCLE ( 'NONE', #10475, 0.3999999999999975797 ) ;
#31706=FACE_BOUND ( 'NONE', #26987, .T. ) ;
#31762=VECTOR ( 'NONE', #36046, 1000.000000000000000 ) ;
#31780=DIRECTION ( 'NONE',  ( -0.000000000000000000, -1.000000000000000000, -0.000000000000000000 ) ) ;
#31784=CARTESIAN_POINT ( 'NONE',  ( -9.424093855413055110, -27.10920654474410796, 54.99999999999997868 ) ) ;
#31786=ORIENTED_EDGE ( 'NONE', *, *, #44375, .F. ) ;
#31787=ADVANCED_FACE ( 'NONE', ( #1764 ), #12687, .T. ) ;
#31789=DIRECTION ( 'NONE',  ( -0.000000000000000000, -1.000000000000000000, -0.000000000000000000 ) ) ;
#31800=TOROIDAL_SURFACE ( 'NONE', #18416, 1.000000000000001332, 0.5000000000000000000 ) ;
#31816=DIRECTION ( 'NONE',  ( 1.000000000000000000, -0.000000000000000000, 2.081668171172170091E-15 ) ) ;
#31835=ORIENTED_EDGE ( 'NONE', *, *, #30757, .T. ) ;
#31849=ORIENTED_EDGE ( 'NONE', *, *, #26187, .T. ) ;
#31873=DIRECTION ( 'NONE',  ( 0.000000000000000000, 1.000000000000000000, -0.000000000000000000 ) ) ;
#31880=EDGE_CURVE ( 'NONE', #4125, #11393, #18976, .T. ) ;
#31886=CARTESIAN_POINT ( 'NONE',  ( -17.79490377976783932, -14.65920654474411045, 52.21286476528345588 ) ) ;
#31900=CIRCLE ( 'NONE', #34234, 1.050000000000002265 ) ;
#31904=EDGE_CURVE ( 'NONE', #30602, #37234, #9583, .T. ) ;
#31915=DIRECTION ( 'NONE',  ( -0.000000000000000000, 0.000000000000000000, 1.000000000000000000 ) ) ;
#31937=CARTESIAN_POINT ( 'NONE',  ( -8.424093855413053333, -25.10920654474410441, 47.99999999999998579 ) ) ;
#31979=ORIENTED_EDGE ( 'NONE', *, *, #31984, .T. ) ;
#31980=DIRECTION ( 'NONE',  ( -1.000000000000000000, 0.000000000000000000, 0.000000000000000000 ) ) ;
#31984=EDGE_CURVE ( 'NONE', #17425, #17144, #28593, .T. ) ;
#32014=DIRECTION ( 'NONE',  ( -0.1240347345892083841, 0.000000000000000000, -0.9922778767136676281 ) ) ;
#32023=DIRECTION ( 'NONE',  ( -0.000000000000000000, -1.000000000000000000, 0.000000000000000000 ) ) ;
#32039=DIRECTION ( 'NONE',  ( -1.000000000000000000, 0.000000000000000000, 0.000000000000000000 ) ) ;
#32067=LINE ( 'NONE', #13089, #25073 ) ;
#32088=VECTOR ( 'NONE', #36178, 1000.000000000000000 ) ;
#32089=DIRECTION ( 'NONE',  ( -0.000000000000000000, -1.000000000000000000, -0.000000000000000000 ) ) ;
#32092=ORIENTED_EDGE ( 'NONE', *, *, #40165, .F. ) ;
#32108=AXIS2_PLACEMENT_3D ( 'NONE', #5070, #46184, #35335 ) ;
#32124=ORIENTED_EDGE ( 'NONE', *, *, #7641, .F. ) ;
#32127=DIRECTION ( 'NONE',  ( -0.000000000000000000, -1.000000000000000000, -0.000000000000000000 ) ) ;
#32140=CARTESIAN_POINT ( 'NONE',  ( -26.92409385541305511, -6.359206544744109735, 63.99999999999998579 ) ) ;
#32144=VECTOR ( 'NONE', #31303, 1000.000000000000000 ) ;
#32155=AXIS2_PLACEMENT_3D ( 'NONE', #16842, #17332, #20801 ) ;
#32160=ORIENTED_EDGE ( 'NONE', *, *, #33, .F. ) ;
#32178=VECTOR ( 'NONE', #5315, 1000.000000000000000 ) ;
#32195=CARTESIAN_POINT ( 'NONE',  ( -4.424093855413056886, -8.109206544744111511, 51.75000000000000000 ) ) ;
#32238=DIRECTION ( 'NONE',  ( 2.081668171172170091E-15, -0.000000000000000000, -1.000000000000000000 ) ) ;
#32250=CIRCLE ( 'NONE', #44837, 1.250000000000001110 ) ;
#32260=AXIS2_PLACEMENT_3D ( 'NONE', #38123, #46019, #18936 ) ;
#32270=DIRECTION ( 'NONE',  ( 0.000000000000000000, 1.000000000000000000, 0.000000000000000000 ) ) ;
#32297=AXIS2_PLACEMENT_3D ( 'NONE', #7977, #4750, #8696 ) ;
#32300=EDGE_LOOP ( 'NONE', ( #32368, #42484 ) ) ;
#32301=LINE ( 'NONE', #35726, #1338 ) ;
#32365=VERTEX_POINT ( 'NONE', #21861 ) ;
#32367=DIRECTION ( 'NONE',  ( 0.000000000000000000, 0.000000000000000000, -1.000000000000000000 ) ) ;
#32368=ORIENTED_EDGE ( 'NONE', *, *, #20631, .T. ) ;
#32385=VECTOR ( 'NONE', #10692, 1000.000000000000000 ) ;
#32412=EDGE_CURVE ( 'NONE', #37238, #10228, #29246, .T. ) ;
#32444=EDGE_CURVE ( 'NONE', #744, #33284, #27668, .T. ) ;
#32461=EDGE_CURVE ( 'NONE', #18891, #13748, #5104, .T. ) ;
#32488=DIRECTION ( 'NONE',  ( 1.000000000000000000, 0.000000000000000000, 0.000000000000000000 ) ) ;
#32490=DIRECTION ( 'NONE',  ( -2.081668171172170091E-15, 0.000000000000000000, 1.000000000000000000 ) ) ;
#32521=DIRECTION ( 'NONE',  ( 2.181982678098338148E-16, 0.000000000000000000, -1.000000000000000000 ) ) ;
#32545=ORIENTED_EDGE ( 'NONE', *, *, #32584, .F. ) ;
#32561=FACE_OUTER_BOUND ( 'NONE', #42761, .T. ) ;
#32584=EDGE_CURVE ( 'NONE', #20093, #24954, #27977, .T. ) ;
#32642=DIRECTION ( 'NONE',  ( 0.000000000000000000, 0.000000000000000000, 1.000000000000000000 ) ) ;
#32656=ORIENTED_EDGE ( 'NONE', *, *, #21722, .T. ) ;
#32660=AXIS2_PLACEMENT_3D ( 'NONE', #34076, #5031, #11680 ) ;
#32688=ORIENTED_EDGE ( 'NONE', *, *, #45240, .F. ) ;
#32705=LINE ( 'NONE', #17451, #44842 ) ;
#32706=EDGE_LOOP ( 'NONE', ( #14644, #20702, #12137, #21825, #5416, #22489, #14970, #34290 ) ) ;
#32720=CARTESIAN_POINT ( 'NONE',  ( -7.924093855413070209, -6.359206544744109735, 52.99999999999997868 ) ) ;
#32791=DIRECTION ( 'NONE',  ( 0.1240347345892083841, 0.000000000000000000, 0.9922778767136676281 ) ) ;
#32801=CARTESIAN_POINT ( 'NONE',  ( -7.424093855413048892, -27.10920654474410796, 77.00000000000000000 ) ) ;
#32812=DIRECTION ( 'NONE',  ( -0.000000000000000000, -1.000000000000000000, -0.000000000000000000 ) ) ;
#32827=ORIENTED_EDGE ( 'NONE', *, *, #40704, .T. ) ;
#32831=VECTOR ( 'NONE', #32127, 1000.000000000000000 ) ;
#32841=ORIENTED_EDGE ( 'NONE', *, *, #40454, .F. ) ;
#32918=EDGE_CURVE ( 'NONE', #26269, #27788, #46884, .T. ) ;
#32926=VECTOR ( 'NONE', #823, 1000.000000000000000 ) ;
#32952=AXIS2_PLACEMENT_3D ( 'NONE', #47025, #24391, #42628 ) ;
#32969=EDGE_CURVE ( 'NONE', #11779, #17527, #31691, .T. ) ;
#33001=DIRECTION ( 'NONE',  ( 0.000000000000000000, 0.000000000000000000, 1.000000000000000000 ) ) ;
#33039=ORIENTED_EDGE ( 'NONE', *, *, #12735, .F. ) ;
#33059=CARTESIAN_POINT ( 'NONE',  ( -17.42409385541305511, -14.80920654474410725, 52.21286476528345588 ) ) ;
#33080=VERTEX_POINT ( 'NONE', #45380 ) ;
#33082=ORIENTED_EDGE ( 'NONE', *, *, #47622, .T. ) ;
#33087=CIRCLE ( 'NONE', #39417, 0.5000000000000004441 ) ;
#33088=ORIENTED_EDGE ( 'NONE', *, *, #28826, .T. ) ;
#33092=DIRECTION ( 'NONE',  ( 0.000000000000000000, 1.000000000000000000, -0.000000000000000000 ) ) ;
#33093=AXIS2_PLACEMENT_3D ( 'NONE', #34704, #12295, #27075 ) ;
#33113=CARTESIAN_POINT ( 'NONE',  ( -6.424093855413055110, -6.359206544744109735, 47.99999999999998579 ) ) ;
#33219=ORIENTED_EDGE ( 'NONE', *, *, #3273, .F. ) ;
#33271=DIRECTION ( 'NONE',  ( 0.000000000000000000, 0.000000000000000000, 1.000000000000000000 ) ) ;
#33284=VERTEX_POINT ( 'NONE', #27451 ) ;
#33290=LINE ( 'NONE', #24969, #27495 ) ;
#33312=LINE ( 'NONE', #37017, #10047 ) ;
#33345=FACE_BOUND ( 'NONE', #35594, .T. ) ;
#33356=DIRECTION ( 'NONE',  ( 1.927470528863119542E-16, 0.000000000000000000, -1.000000000000000000 ) ) ;
#33377=AXIS2_PLACEMENT_3D ( 'NONE', #41792, #27246, #19615 ) ;
#33383=LINE ( 'NONE', #25779, #46940 ) ;
#33387=EDGE_CURVE ( 'NONE', #3383, #43409, #43211, .T. ) ;
#33392=EDGE_LOOP ( 'NONE', ( #38368, #17363, #20734, #48450, #5381, #46885, #19453, #46791, #19619, #33219 ) ) ;
#33413=CYLINDRICAL_SURFACE ( 'NONE', #45632, 2.000000000000001776 ) ;
#33446=DIRECTION ( 'NONE',  ( 0.000000000000000000, 0.000000000000000000, -1.000000000000000000 ) ) ;
#33447=AXIS2_PLACEMENT_3D ( 'NONE', #27186, #11934, #41970 ) ;
#33458=DIRECTION ( 'NONE',  ( 0.000000000000000000, 1.000000000000000000, -0.000000000000000000 ) ) ;
#33472=EDGE_LOOP ( 'NONE', ( #25268, #30216, #23187, #15542 ) ) ;
#33531=CARTESIAN_POINT ( 'NONE',  ( -6.424093855413055110, -25.10920654474410441, 45.99999999999998579 ) ) ;
#33538=DIRECTION ( 'NONE',  ( -0.000000000000000000, -1.000000000000000000, -0.000000000000000000 ) ) ;
#33549=LINE ( 'NONE', #36756, #36440 ) ;
#33550=AXIS2_PLACEMENT_3D ( 'NONE', #36364, #2645, #10527 ) ;
#33572=CARTESIAN_POINT ( 'NONE',  ( -7.924093855413066656, -6.859206544744110623, 52.99999999999997868 ) ) ;
#33606=ORIENTED_EDGE ( 'NONE', *, *, #21745, .T. ) ;
#33607=DIRECTION ( 'NONE',  ( 1.000000000000000000, 0.000000000000000000, -2.406186529621654018E-16 ) ) ;
#33615=AXIS2_PLACEMENT_3D ( 'NONE', #27985, #10004, #40047 ) ;
#33625=VECTOR ( 'NONE', #15139, 1000.000000000000000 ) ;
#33697=LINE ( 'NONE', #487, #47002 ) ;
#33698=DIRECTION ( 'NONE',  ( 1.000000000000000000, 0.000000000000000000, 0.000000000000000000 ) ) ;
#33699=VECTOR ( 'NONE', #48411, 1000.000000000000000 ) ;
#33702=ORIENTED_EDGE ( 'NONE', *, *, #9495, .T. ) ;
#33703=ORIENTED_EDGE ( 'NONE', *, *, #38701, .F. ) ;
#33748=DIRECTION ( 'NONE',  ( 1.000000000000000000, 0.000000000000000000, -5.466375705775733989E-17 ) ) ;
#33756=CARTESIAN_POINT ( 'NONE',  ( -27.42409385541305511, -27.10920654474410796, 54.99999999999997868 ) ) ;
#33759=CYLINDRICAL_SURFACE ( 'NONE', #6164, 0.5000000000000004441 ) ;
#33767=VERTEX_POINT ( 'NONE', #27876 ) ;
#33775=ADVANCED_FACE ( 'NONE', ( #47334 ), #46362, .F. ) ;
#33786=ORIENTED_EDGE ( 'NONE', *, *, #28521, .T. ) ;
#33787=APPLICATION_CONTEXT ( 'automotive_design' ) ;
#33805=DIRECTION ( 'NONE',  ( 1.927470528863119542E-16, 0.000000000000000000, -1.000000000000000000 ) ) ;
#33834=DIRECTION ( 'NONE',  ( 0.000000000000000000, 0.000000000000000000, -1.000000000000000000 ) ) ;
#33839=EDGE_CURVE ( 'NONE', #42725, #4116, #2505, .T. ) ;
#33862=DIRECTION ( 'NONE',  ( 0.000000000000000000, 0.000000000000000000, 1.000000000000000000 ) ) ;
#33893=ORIENTED_EDGE ( 'NONE', *, *, #25095, .F. ) ;
#33908=AXIS2_PLACEMENT_3D ( 'NONE', #34345, #23781, #38534 ) ;
#33921=VECTOR ( 'NONE', #3088, 1000.000000000000000 ) ;
#33933=ORIENTED_EDGE ( 'NONE', *, *, #38444, .T. ) ;
#33952=ORIENTED_EDGE ( 'NONE', *, *, #20631, .F. ) ;
#33988=DIRECTION ( 'NONE',  ( 0.000000000000000000, 1.000000000000000000, -0.000000000000000000 ) ) ;
#34076=CARTESIAN_POINT ( 'NONE',  ( -20.92409385541305511, -25.10920654474410441, 80.49999999999998579 ) ) ;
#34106=CYLINDRICAL_SURFACE ( 'NONE', #22139, 0.5000000000000004441 ) ;
#34110=FACE_OUTER_BOUND ( 'NONE', #2784, .T. ) ;
#34123=CARTESIAN_POINT ( 'NONE',  ( -15.92409385541305333, -15.80920654474410725, 48.99999999999997868 ) ) ;
#34146=ORIENTED_EDGE ( 'NONE', *, *, #29042, .T. ) ;
#34162=FACE_OUTER_BOUND ( 'NONE', #18321, .T. ) ;
#34174=ORIENTED_EDGE ( 'NONE', *, *, #36337, .F. ) ;
#34231=ORIENTED_EDGE ( 'NONE', *, *, #33, .T. ) ;
#34234=AXIS2_PLACEMENT_3D ( 'NONE', #4300, #23258, #34564 ) ;
#34253=( NAMED_UNIT ( * ) SI_UNIT ( $, .STERADIAN. ) SOLID_ANGLE_UNIT ( ) );
#34265=CARTESIAN_POINT ( 'NONE',  ( -46.92409385541305511, -17.80920654474410370, 61.49999999999999289 ) ) ;
#34275=ORIENTED_EDGE ( 'NONE', *, *, #26167, .F. ) ;
#34280=EDGE_CURVE ( 'NONE', #9420, #40683, #2616, .T. ) ;
#34290=ORIENTED_EDGE ( 'NONE', *, *, #20587, .T. ) ;
#34311=DIRECTION ( 'NONE',  ( 1.000000000000000000, 0.000000000000000000, 0.000000000000000000 ) ) ;
#34319=ORIENTED_EDGE ( 'NONE', *, *, #13591, .F. ) ;
#34345=CARTESIAN_POINT ( 'NONE',  ( -45.92409385541305511, -17.80920654474410370, 70.50000000000000000 ) ) ;
#34349=DIRECTION ( 'NONE',  ( 0.000000000000000000, 1.000000000000000000, -0.000000000000000000 ) ) ;
#34418=ADVANCED_FACE ( 'NONE', ( #34110 ), #41765, .T. ) ;
#34442=ORIENTED_EDGE ( 'NONE', *, *, #40191, .F. ) ;
#34471=VECTOR ( 'NONE', #45171, 1000.000000000000000 ) ;
#34473=CARTESIAN_POINT ( 'NONE',  ( -33.52409385541305653, -2.423472813913224222, 52.29999999999998295 ) ) ;
#34501=EDGE_CURVE ( 'NONE', #9962, #23568, #39024, .T. ) ;
#34523=AXIS2_PLACEMENT_3D ( 'NONE', #35391, #33988, #46498 ) ;
#34564=DIRECTION ( 'NONE',  ( 0.000000000000000000, 0.000000000000000000, -1.000000000000000000 ) ) ;
#34577=LINE ( 'NONE', #39008, #35427 ) ;
#34582=CARTESIAN_POINT ( 'NONE',  ( -50.42409385541304800, -25.10920654474410441, 56.99999999999999289 ) ) ;
#34584=EDGE_LOOP ( 'NONE', ( #39499, #31084, #15400, #42862 ) ) ;
#34585=DIRECTION ( 'NONE',  ( 0.000000000000000000, 0.000000000000000000, 1.000000000000000000 ) ) ;
#34626=CIRCLE ( 'NONE', #15737, 0.5000000000000004441 ) ;
#34630=EDGE_CURVE ( 'NONE', #31526, #3895, #33549, .T. ) ;
#34634=AXIS2_PLACEMENT_3D ( 'NONE', #1371, #12938, #28216 ) ;
#34646=EDGE_LOOP ( 'NONE', ( #23001, #8170, #23013, #11606 ) ) ;
#34652=VERTEX_POINT ( 'NONE', #43958 ) ;
#34660=AXIS2_PLACEMENT_3D ( 'NONE', #6501, #36503, #2785 ) ;
#34669=VERTEX_POINT ( 'NONE', #44207 ) ;
#34671=AXIS2_PLACEMENT_3D ( 'NONE', #68, #38439, #43796 ) ;
#34678=VECTOR ( 'NONE', #43882, 1000.000000000000000 ) ;
#34693=( NAMED_UNIT ( * ) SI_UNIT ( $, .STERADIAN. ) SOLID_ANGLE_UNIT ( ) );
#34704=CARTESIAN_POINT ( 'NONE',  ( -46.92409385541305511, -17.80920654474410370, 61.49999999999999289 ) ) ;
#34722=VECTOR ( 'NONE', #40040, 1000.000000000000000 ) ;
#34828=ORIENTED_EDGE ( 'NONE', *, *, #24945, .F. ) ;
#34831=DIRECTION ( 'NONE',  ( -0.000000000000000000, -1.000000000000000000, 0.000000000000000000 ) ) ;
#34874=ORIENTED_EDGE ( 'NONE', *, *, #7641, .T. ) ;
#34882=DIRECTION ( 'NONE',  ( 0.000000000000000000, 0.000000000000000000, 1.000000000000000000 ) ) ;
#34888=DIRECTION ( 'NONE',  ( -9.637352644315596475E-17, 0.000000000000000000, -1.000000000000000000 ) ) ;
#34895=ORIENTED_EDGE ( 'NONE', *, *, #16754, .T. ) ;
#34944=VECTOR ( 'NONE', #17534, 1000.000000000000000 ) ;
#34960=ADVANCED_FACE ( 'NONE', ( #31588 ), #3449, .T. ) ;
#34970=VERTEX_POINT ( 'NONE', #24202 ) ;
#35016=DIRECTION ( 'NONE',  ( 2.081668171172170091E-15, 0.000000000000000000, -1.000000000000000000 ) ) ;
#35038=ORIENTED_EDGE ( 'NONE', *, *, #22508, .F. ) ;
#35054=ORIENTED_EDGE ( 'NONE', *, *, #46589, .F. ) ;
#35058=PRODUCT_DEFINITION_SHAPE ( 'NONE', 'NONE',  #29471 ) ;
#35084=PLANE ( 'NONE',  #32108 ) ;
#35090=CARTESIAN_POINT ( 'NONE',  ( -7.924093855413070209, -6.359206544744109735, 52.99999999999997868 ) ) ;
#35105=ORIENTED_EDGE ( 'NONE', *, *, #2535, .T. ) ;
#35119=ORIENTED_EDGE ( 'NONE', *, *, #35910, .F. ) ;
#35123=CARTESIAN_POINT ( 'NONE',  ( -48.42409385541304800, -25.10920654474410441, 79.99999999999998579 ) ) ;
#35125=AXIS2_PLACEMENT_3D ( 'NONE', #28236, #43266, #15925 ) ;
#35146=PRODUCT_DEFINITION_CONTEXT ( 'detailed design', #43887, 'design' ) ;
#35150=ORIENTED_EDGE ( 'NONE', *, *, #22218, .T. ) ;
#35203=DIRECTION ( 'NONE',  ( 0.000000000000000000, 1.000000000000000000, -0.000000000000000000 ) ) ;
#35213=ORIENTED_EDGE ( 'NONE', *, *, #35717, .T. ) ;
#35219=FACE_OUTER_BOUND ( 'NONE', #6392, .T. ) ;
#35246=AXIS2_PLACEMENT_3D ( 'NONE', #837, #46133, #26447 ) ;
#35253=EDGE_LOOP ( 'NONE', ( #7987, #40459, #48125, #40785 ) ) ;
#35256=PLANE ( 'NONE',  #41516 ) ;
#35261=AXIS2_PLACEMENT_3D ( 'NONE', #38326, #12012, #8318 ) ;
#35278=CARTESIAN_POINT ( 'NONE',  ( -35.32409385541306079, -6.359206544744109735, 52.29999999999998295 ) ) ;
#35314=EDGE_CURVE ( 'NONE', #26221, #43409, #4953, .T. ) ;
#35322=EDGE_CURVE ( 'NONE', #37238, #31278, #17934, .T. ) ;
#35335=DIRECTION ( 'NONE',  ( -0.1240347345892083702, 0.000000000000000000, -0.9922778767136676281 ) ) ;
#35355=CARTESIAN_POINT ( 'NONE',  ( -50.42409385541304800, -25.10920654474410441, 63.99999999999998579 ) ) ;
#35357=ORIENTED_EDGE ( 'NONE', *, *, #24957, .T. ) ;
#35391=CARTESIAN_POINT ( 'NONE',  ( -27.42409385541305511, -25.10920654474410441, 63.99999999999998579 ) ) ;
#35402=ORIENTED_EDGE ( 'NONE', *, *, #16023, .F. ) ;
#35427=VECTOR ( 'NONE', #42473, 1000.000000000000000 ) ;
#35466=CIRCLE ( 'NONE', #29184, 1.250000000000007994 ) ;
#35495=CARTESIAN_POINT ( 'NONE',  ( -48.42409385541304800, -25.10920654474410441, 47.99999999999998579 ) ) ;
#35506=DIRECTION ( 'NONE',  ( 0.000000000000000000, 0.000000000000000000, 1.000000000000000000 ) ) ;
#35517=DIRECTION ( 'NONE',  ( 0.000000000000000000, 0.000000000000000000, -1.000000000000000000 ) ) ;
#35523=DIRECTION ( 'NONE',  ( 0.000000000000000000, 1.000000000000000000, 0.000000000000000000 ) ) ;
#35527=LINE ( 'NONE', #2528, #34944 ) ;
#35529=CYLINDRICAL_SURFACE ( 'NONE', #23463, 0.3999999999999975797 ) ;
#35538=CIRCLE ( 'NONE', #4096, 1.500000000000001332 ) ;
#35571=DIRECTION ( 'NONE',  ( -0.000000000000000000, -1.000000000000000000, -0.000000000000000000 ) ) ;
#35588=DIRECTION ( 'NONE',  ( -1.000000000000000000, 0.000000000000000000, 0.000000000000000000 ) ) ;
#35593=ADVANCED_FACE ( 'NONE', ( #12757 ), #31800, .T. ) ;
#35594=EDGE_LOOP ( 'NONE', ( #29717, #1275, #43394, #41590, #1928, #15116, #12604, #13884 ) ) ;
#35602=ORIENTED_EDGE ( 'NONE', *, *, #18831, .F. ) ;
#35631=DIRECTION ( 'NONE',  ( -1.000000000000000000, 0.000000000000000000, 0.000000000000000000 ) ) ;
#35689=DIRECTION ( 'NONE',  ( -1.000000000000000000, 0.000000000000000000, 9.637352644315596475E-17 ) ) ;
#35698=ORIENTED_EDGE ( 'NONE', *, *, #36572, .F. ) ;
#35706=ORIENTED_EDGE ( 'NONE', *, *, #2306, .T. ) ;
#35717=EDGE_CURVE ( 'NONE', #43808, #19690, #43536, .T. ) ;
#35726=CARTESIAN_POINT ( 'NONE',  ( -33.52409385541305653, -6.359206544744109735, 52.29999999999998295 ) ) ;
#35729=VERTEX_POINT ( 'NONE', #44030 ) ;
#35746=CARTESIAN_POINT ( 'NONE',  ( -28.42409385541305511, -6.359206544744109735, 47.99999999999997868 ) ) ;
#35759=EDGE_CURVE ( 'NONE', #3842, #34970, #28671, .T. ) ;
#35774=CARTESIAN_POINT ( 'NONE',  ( -6.424093855413055110, -25.10920654474410441, 47.99999999999998579 ) ) ;
#35786=CARTESIAN_POINT ( 'NONE',  ( -17.42409385541305511, -14.80920654474410725, 48.99999999999997868 ) ) ;
#35795=ORIENTED_EDGE ( 'NONE', *, *, #40165, .T. ) ;
#35870=DIRECTION ( 'NONE',  ( 0.000000000000000000, 1.000000000000000000, -0.000000000000000000 ) ) ;
#35883=CARTESIAN_POINT ( 'NONE',  ( -43.14308517176575464, -27.10920654474410796, 57.24806946917839667 ) ) ;
#35910=EDGE_CURVE ( 'NONE', #36791, #45046, #35527, .T. ) ;
#35919=ORIENTED_EDGE ( 'NONE', *, *, #1037, .T. ) ;
#35926=CIRCLE ( 'NONE', #19450, 2.000000000000001776 ) ;
#35931=CARTESIAN_POINT ( 'NONE',  ( -27.42409385541305511, -25.10920654474410441, 45.99999999999998579 ) ) ;
#35944=DIRECTION ( 'NONE',  ( 1.000000000000000000, 0.000000000000000000, 0.000000000000000000 ) ) ;
#35953=ORIENTED_EDGE ( 'NONE', *, *, #47687, .F. ) ;
#35978=EDGE_CURVE ( 'NONE', #30260, #7661, #14301, .T. ) ;
#36000=CARTESIAN_POINT ( 'NONE',  ( -43.17409385541305511, -25.10920654474410441, 56.99999999999999289 ) ) ;
#36004=DIRECTION ( 'NONE',  ( 1.927470528863119542E-16, 0.000000000000000000, -1.000000000000000000 ) ) ;
#36016=VERTEX_POINT ( 'NONE', #25649 ) ;
#36021=CIRCLE ( 'NONE', #9293, 1.000000000000000888 ) ;
#36023=VECTOR ( 'NONE', #24324, 1000.000000000000000 ) ;
#36029=FACE_OUTER_BOUND ( 'NONE', #1668, .T. ) ;
#36046=DIRECTION ( 'NONE',  ( -0.000000000000000000, 1.000000000000000000, -0.000000000000000000 ) ) ;
#36050=EDGE_CURVE ( 'NONE', #41929, #8183, #18450, .T. ) ;
#36071=CARTESIAN_POINT ( 'NONE',  ( -27.42409385541305156, -14.65920654474411045, 52.21286476528344878 ) ) ;
#36080=AXIS2_PLACEMENT_3D ( 'NONE', #43069, #25331, #47499 ) ;
#36122=VECTOR ( 'NONE', #40822, 1000.000000000000000 ) ;
#36148=CYLINDRICAL_SURFACE ( 'NONE', #36080, 1.250000000000001110 ) ;
#36150=VECTOR ( 'NONE', #39067, 1000.000000000000000 ) ;
#36162=ORIENTED_EDGE ( 'NONE', *, *, #37407, .F. ) ;
#36163=LINE ( 'NONE', #43588, #8702 ) ;
#36167=EDGE_LOOP ( 'NONE', ( #40167, #38432, #46913, #37653, #8423 ) ) ;
#36178=DIRECTION ( 'NONE',  ( 0.000000000000000000, 1.000000000000000000, -9.912705577010318647E-16 ) ) ;
#36184=DIRECTION ( 'NONE',  ( 1.000000000000000000, 0.000000000000000000, 0.000000000000000000 ) ) ;
#36190=DIRECTION ( 'NONE',  ( -2.081668171172170091E-15, 0.000000000000000000, 1.000000000000000000 ) ) ;
#36199=ADVANCED_FACE ( 'NONE', ( #35219 ), #16739, .F. ) ;
#36226=FACE_OUTER_BOUND ( 'NONE', #16777, .T. ) ;
#36240=DIRECTION ( 'NONE',  ( -1.000000000000000000, 0.000000000000000000, -8.260587980841940012E-17 ) ) ;
#36283=CARTESIAN_POINT ( 'NONE',  ( -33.95962776134579286, -8.109206544744111511, 51.75000000000000711 ) ) ;
#36291=ORIENTED_EDGE ( 'NONE', *, *, #3328, .F. ) ;
#36328=CARTESIAN_POINT ( 'NONE',  ( -46.92409385541305511, -17.80920654474410370, 61.49999999999999289 ) ) ;
#36337=EDGE_CURVE ( 'NONE', #17527, #43029, #14491, .T. ) ;
#36353=VERTEX_POINT ( 'NONE', #11774 ) ;
#36364=CARTESIAN_POINT ( 'NONE',  ( -13.92409385541305511, -10.60920654474410618, 79.49999999999998579 ) ) ;
#36369=CARTESIAN_POINT ( 'NONE',  ( -17.05328393105827089, -14.65920654474411045, 52.21286476528345588 ) ) ;
#36374=EDGE_CURVE ( 'NONE', #23071, #35729, #38930, .T. ) ;
#36398=CARTESIAN_POINT ( 'NONE',  ( -33.52409385541305653, -25.10920654474410441, 48.79999999999998295 ) ) ;
#36436=ORIENTED_EDGE ( 'NONE', *, *, #47403, .F. ) ;
#36440=VECTOR ( 'NONE', #40719, 1000.000000000000114 ) ;
#36460=CARTESIAN_POINT ( 'NONE',  ( -17.05328393105827089, -14.65920654474411045, 47.99999999999998579 ) ) ;
#36477=CARTESIAN_POINT ( 'NONE',  ( -42.07024770156689897, -27.10920654474410796, 65.83076923076922071 ) ) ;
#36503=DIRECTION ( 'NONE',  ( 0.000000000000000000, 0.000000000000000000, -1.000000000000000000 ) ) ;
#36532=EDGE_LOOP ( 'NONE', ( #29841, #11603, #45158, #32545 ) ) ;
#36572=EDGE_CURVE ( 'NONE', #12722, #8993, #22559, .T. ) ;
#36587=EDGE_CURVE ( 'NONE', #115, #3383, #20834, .T. ) ;
#36589=EDGE_LOOP ( 'NONE', ( #42451, #25492, #41888, #39597 ) ) ;
#36656=CARTESIAN_POINT ( 'NONE',  ( -13.92409385541305511, -10.10920654474410618, 79.49999999999998579 ) ) ;
#36714=FACE_OUTER_BOUND ( 'NONE', #25246, .T. ) ;
#36724=ORIENTED_EDGE ( 'NONE', *, *, #37955, .F. ) ;
#36756=CARTESIAN_POINT ( 'NONE',  ( -42.07024770156689897, -25.10920654474410441, 65.83076923076922071 ) ) ;
#36771=EDGE_CURVE ( 'NONE', #24008, #19690, #17525, .T. ) ;
#36779=AXIS2_PLACEMENT_3D ( 'NONE', #26075, #37368, #29765 ) ;
#36791=VERTEX_POINT ( 'NONE', #23181 ) ;
#36797=CARTESIAN_POINT ( 'NONE',  ( -8.424093855413060439, -6.859206544744110623, 47.99999999999998579 ) ) ;
#36815=AXIS2_PLACEMENT_3D ( 'NONE', #1418, #27286, #35631 ) ;
#36848=VECTOR ( 'NONE', #13268, 1000.000000000000000 ) ;
#36951=ORIENTED_EDGE ( 'NONE', *, *, #7644, .T. ) ;
#36977=ORIENTED_EDGE ( 'NONE', *, *, #30706, .T. ) ;
#36980=EDGE_CURVE ( 'NONE', #3895, #7661, #1236, .T. ) ;
#37009=VERTEX_POINT ( 'NONE', #6155 ) ;
#37017=CARTESIAN_POINT ( 'NONE',  ( -20.92409385541305511, -10.60920654474410618, 81.99999999999998579 ) ) ;
#37046=CIRCLE ( 'NONE', #39431, 2.500000000000002220 ) ;
#37060=ORIENTED_EDGE ( 'NONE', *, *, #32584, .T. ) ;
#37066=VERTEX_POINT ( 'NONE', #6398 ) ;
#37075=EDGE_LOOP ( 'NONE', ( #36977, #12728, #45049, #17827 ) ) ;
#37086=EDGE_CURVE ( 'NONE', #33080, #19972, #16970, .T. ) ;
#37098=LINE ( 'NONE', #7830, #9264 ) ;
#37134=EDGE_CURVE ( 'NONE', #4687, #9150, #22383, .T. ) ;
#37146=DIRECTION ( 'NONE',  ( 1.000000000000000000, 0.000000000000000000, 8.260587980841940012E-17 ) ) ;
#37164=CARTESIAN_POINT ( 'NONE',  ( -35.32409385541306079, -6.359206544744109735, 48.79999999999998295 ) ) ;
#37181=CARTESIAN_POINT ( 'NONE',  ( -27.42409385541305511, -15.80920654474410725, 63.99999999999998579 ) ) ;
#37234=VERTEX_POINT ( 'NONE', #37629 ) ;
#37238=VERTEX_POINT ( 'NONE', #14967 ) ;
#37241=ADVANCED_FACE ( 'NONE', ( #22149 ), #29526, .F. ) ;
#37256=ORIENTED_EDGE ( 'NONE', *, *, #40704, .F. ) ;
#37284=AXIS2_PLACEMENT_3D ( 'NONE', #9799, #29469, #18124 ) ;
#37318=CARTESIAN_POINT ( 'NONE',  ( -50.42509385541305988, -8.109206544744111511, 51.54999999999998295 ) ) ;
#37327=DIRECTION ( 'NONE',  ( -0.000000000000000000, 0.000000000000000000, 1.000000000000000000 ) ) ;
#37336=ORIENTED_EDGE ( 'NONE', *, *, #15112, .F. ) ;
#37368=DIRECTION ( 'NONE',  ( -0.000000000000000000, -1.000000000000000000, 0.000000000000000000 ) ) ;
#37378=ORIENTED_EDGE ( 'NONE', *, *, #26839, .F. ) ;
#37397=CARTESIAN_POINT ( 'NONE',  ( -41.15852941833841783, -25.10920654474410441, 56.99999999999997868 ) ) ;
#37407=EDGE_CURVE ( 'NONE', #7384, #11732, #9746, .T. ) ;
#37412=EDGE_LOOP ( 'NONE', ( #2182, #37916, #8787, #22675, #15191 ) ) ;
#37418=FACE_OUTER_BOUND ( 'NONE', #44964, .T. ) ;
#37432=LINE ( 'NONE', #16005, #14845 ) ;
#37463=CIRCLE ( 'NONE', #16224, 1.999999999999994893 ) ;
#37474=EDGE_LOOP ( 'NONE', ( #8497, #41756, #10015, #45896, #24982, #3983, #46090, #15865, #46331, #5769 ) ) ;
#37479=FACE_OUTER_BOUND ( 'NONE', #12593, .T. ) ;
#37496=CIRCLE ( 'NONE', #21794, 1.500000000000001332 ) ;
#37497=CIRCLE ( 'NONE', #548, 1.500000000000001332 ) ;
#37500=EDGE_CURVE ( 'NONE', #42725, #44357, #4280, .T. ) ;
#37509=LINE ( 'NONE', #16806, #26280 ) ;
#37511=ORIENTED_EDGE ( 'NONE', *, *, #38866, .F. ) ;
#37522=DIRECTION ( 'NONE',  ( 0.000000000000000000, 0.000000000000000000, 1.000000000000000000 ) ) ;
#37544=EDGE_CURVE ( 'NONE', #1836, #22645, #28665, .T. ) ;
#37571=ORIENTED_EDGE ( 'NONE', *, *, #96, .T. ) ;
#37587=ORIENTED_EDGE ( 'NONE', *, *, #15293, .T. ) ;
#37608=DIRECTION ( 'NONE',  ( -0.000000000000000000, -1.000000000000000000, -0.000000000000000000 ) ) ;
#37621=CARTESIAN_POINT ( 'NONE',  ( -27.42409385541305156, -14.65920654474411045, 47.99999999999997868 ) ) ;
#37629=CARTESIAN_POINT ( 'NONE',  ( -14.92409385541305333, -14.80920654474410725, 79.00000000000000000 ) ) ;
#37634=VECTOR ( 'NONE', #27647, 1000.000000000000000 ) ;
#37637=DIRECTION ( 'NONE',  ( 0.000000000000000000, 0.000000000000000000, 1.000000000000000000 ) ) ;
#37647=SHAPE_REPRESENTATION_RELATIONSHIP ( 'NONE' , 'NONE' ,  #46513, #12638 ) ;
#37653=ORIENTED_EDGE ( 'NONE', *, *, #8028, .F. ) ;
#37680=CARTESIAN_POINT ( 'NONE',  ( -17.05328393105827089, -14.65920654474411045, 48.99999999999997868 ) ) ;
#37686=EDGE_LOOP ( 'NONE', ( #18479, #38113, #39811, #5784, #13207, #38863, #6197, #41878 ) ) ;
#37696=ORIENTED_EDGE ( 'NONE', *, *, #226, .T. ) ;
#37709=EDGE_CURVE ( 'NONE', #20623, #22645, #37509, .T. ) ;
#37726=AXIS2_PLACEMENT_3D ( 'NONE', #4636, #4393, #15948 ) ;
#37744=FACE_OUTER_BOUND ( 'NONE', #912, .T. ) ;
#37758=LINE ( 'NONE', #18810, #11933 ) ;
#37794=DIRECTION ( 'NONE',  ( 0.000000000000000000, 0.000000000000000000, 1.000000000000000000 ) ) ;
#37795=VERTEX_POINT ( 'NONE', #39478 ) ;
#37856=VECTOR ( 'NONE', #39223, 1000.000000000000000 ) ;
#37916=ORIENTED_EDGE ( 'NONE', *, *, #36050, .T. ) ;
#37923=EDGE_LOOP ( 'NONE', ( #17081, #25511, #5628, #21575, #31453 ) ) ;
#37955=EDGE_CURVE ( 'NONE', #33080, #31526, #9924, .T. ) ;
#37966=FACE_OUTER_BOUND ( 'NONE', #32300, .T. ) ;
#37998=DIRECTION ( 'NONE',  ( 0.000000000000000000, 1.000000000000000000, -0.000000000000000000 ) ) ;
#37999=CARTESIAN_POINT ( 'NONE',  ( -4.924093855413054222, -6.859206544744110623, 63.99999999999998579 ) ) ;
#38021=CARTESIAN_POINT ( 'NONE',  ( -43.14308517176575464, -25.10920654474410441, 57.24806946917839667 ) ) ;
#38029=FACE_OUTER_BOUND ( 'NONE', #5713, .T. ) ;
#38036=EDGE_CURVE ( 'NONE', #37009, #45418, #19978, .T. ) ;
#38049=PRODUCT_CONTEXT ( 'NONE', #33787, 'mechanical' ) ;
#38064=ADVANCED_FACE ( 'NONE', ( #47044 ), #8904, .T. ) ;
#38065=VERTEX_POINT ( 'NONE', #13050 ) ;
#38075=ORIENTED_EDGE ( 'NONE', *, *, #41984, .T. ) ;
#38113=ORIENTED_EDGE ( 'NONE', *, *, #11237, .F. ) ;
#38116=CARTESIAN_POINT ( 'NONE',  ( -15.92409385541305333, -15.80920654474410725, 52.21286476528345588 ) ) ;
#38121=EDGE_LOOP ( 'NONE', ( #23549, #35213, #23426, #4663, #42687, #40423, #47719, #35698, #6259, #13947, #37587, #23043, #14117, #18119 ) ) ;
#38123=CARTESIAN_POINT ( 'NONE',  ( -27.42409385541305511, -25.10920654474410441, 81.99999999999998579 ) ) ;
#38147=DIRECTION ( 'NONE',  ( -5.466375705775733989E-17, 0.000000000000000000, -1.000000000000000000 ) ) ;
#38171=CARTESIAN_POINT ( 'NONE',  ( -48.42409385541304800, -25.10920654474410441, 47.99999999999998579 ) ) ;
#38185=DIRECTION ( 'NONE',  ( 0.000000000000000000, 0.000000000000000000, 1.000000000000000000 ) ) ;
#38202=AXIS2_PLACEMENT_3D ( 'NONE', #1443, #28288, #16699 ) ;
#38208=DIRECTION ( 'NONE',  ( 0.000000000000000000, 0.000000000000000000, -1.000000000000000000 ) ) ;
#38219=DIRECTION ( 'NONE',  ( 0.000000000000000000, 9.912705577010318647E-16, 1.000000000000000000 ) ) ;
#38231=LINE ( 'NONE', #19296, #9275 ) ;
#38242=VECTOR ( 'NONE', #12835, 1000.000000000000000 ) ;
#38326=CARTESIAN_POINT ( 'NONE',  ( -26.92409385541305511, -6.859206544744110623, 47.99999999999997868 ) ) ;
#38327=LINE ( 'NONE', #16411, #39793 ) ;
#38331=VECTOR ( 'NONE', #29939, 1000.000000000000000 ) ;
#38333=DIRECTION ( 'NONE',  ( 0.000000000000000000, 0.000000000000000000, -1.000000000000000000 ) ) ;
#38343=ADVANCED_FACE ( 'NONE', ( #16448 ), #31004, .T. ) ;
#38368=ORIENTED_EDGE ( 'NONE', *, *, #23943, .F. ) ;
#38373=AXIS2_PLACEMENT_3D ( 'NONE', #17336, #9244, #1848 ) ;
#38389=DIRECTION ( 'NONE',  ( -1.000000000000000000, 0.000000000000000000, 5.466375705775733989E-17 ) ) ;
#38407=COLOUR_RGB ( '', 0.31764706, 0.68627451, 0.89019608) ;
#38412=AXIS2_PLACEMENT_3D ( 'NONE', #43666, #46863, #17036 ) ;
#38432=ORIENTED_EDGE ( 'NONE', *, *, #26119, .F. ) ;
#38439=DIRECTION ( 'NONE',  ( 0.000000000000000000, 1.000000000000000000, 0.000000000000000000 ) ) ;
#38444=EDGE_CURVE ( 'NONE', #28641, #25463, #44279, .T. ) ;
#38474=DIRECTION ( 'NONE',  ( 0.000000000000000000, 0.000000000000000000, -1.000000000000000000 ) ) ;
#38478=DIRECTION ( 'NONE',  ( 1.927470528863119542E-16, 0.000000000000000000, -1.000000000000000000 ) ) ;
#38479=CARTESIAN_POINT ( 'NONE',  ( -6.424093855413055110, -25.10920654474410441, 45.99999999999998579 ) ) ;
#38484=DIRECTION ( 'NONE',  ( 8.260587980841940012E-17, 0.000000000000000000, -1.000000000000000000 ) ) ;
#38493=VERTEX_POINT ( 'NONE', #43306 ) ;
#38502=AXIS2_PLACEMENT_3D ( 'NONE', #9629, #32270, #12813 ) ;
#38503=DIRECTION ( 'NONE',  ( -9.637352644315596475E-17, 0.000000000000000000, -1.000000000000000000 ) ) ;
#38534=DIRECTION ( 'NONE',  ( 0.000000000000000000, 0.000000000000000000, 1.000000000000000000 ) ) ;
#38541=CARTESIAN_POINT ( 'NONE',  ( -27.42409385541305156, -14.65920654474411045, 47.99999999999997868 ) ) ;
#38585=CIRCLE ( 'NONE', #11886, 2.500000000000000444 ) ;
#38589=ORIENTED_EDGE ( 'NONE', *, *, #31325, .F. ) ;
#38626=ORIENTED_EDGE ( 'NONE', *, *, #6199, .F. ) ;
#38637=ORIENTED_EDGE ( 'NONE', *, *, #27465, .T. ) ;
#38652=VERTEX_POINT ( 'NONE', #12937 ) ;
#38685=DIRECTION ( 'NONE',  ( 3.652049423109068320E-16, -0.000000000000000000, 1.000000000000000000 ) ) ;
#38701=EDGE_CURVE ( 'NONE', #5342, #39291, #12226, .T. ) ;
#38718=EDGE_CURVE ( 'NONE', #16341, #2752, #16871, .T. ) ;
#38748=ORIENTED_EDGE ( 'NONE', *, *, #23395, .F. ) ;
#38753=DIRECTION ( 'NONE',  ( 0.000000000000000000, 0.000000000000000000, 1.000000000000000000 ) ) ;
#38860=CARTESIAN_POINT ( 'NONE',  ( -29.92409385541305156, -6.859206544744110623, 63.99999999999998579 ) ) ;
#38863=ORIENTED_EDGE ( 'NONE', *, *, #37955, .T. ) ;
#38866=EDGE_CURVE ( 'NONE', #14458, #17537, #22967, .T. ) ;
#38888=VECTOR ( 'NONE', #26899, 1000.000000000000000 ) ;
#38930=CIRCLE ( 'NONE', #9064, 2.000000000000001776 ) ;
#39000=CYLINDRICAL_SURFACE ( 'NONE', #16199, 1.500000000000001332 ) ;
#39008=CARTESIAN_POINT ( 'NONE',  ( -33.52409385541305653, -6.359206544744109735, 48.79999999999998295 ) ) ;
#39010=ORIENTED_EDGE ( 'NONE', *, *, #3826, .T. ) ;
#39020=DIRECTION ( 'NONE',  ( -1.000000000000000000, 0.000000000000000000, 0.000000000000000000 ) ) ;
#39024=LINE ( 'NONE', #24985, #31762 ) ;
#39049=LINE ( 'NONE', #46211, #14951 ) ;
#39064=ORIENTED_EDGE ( 'NONE', *, *, #3947, .F. ) ;
#39067=DIRECTION ( 'NONE',  ( 1.000000000000000000, -0.000000000000000000, -0.000000000000000000 ) ) ;
#39076=CARTESIAN_POINT ( 'NONE',  ( -6.424093855413055110, -25.10920654474410441, 47.99999999999998579 ) ) ;
#39079=LINE ( 'NONE', #9060, #20296 ) ;
#39093=CIRCLE ( 'NONE', #10764, 1.250000000000001110 ) ;
#39109=ORIENTED_EDGE ( 'NONE', *, *, #4312, .F. ) ;
#39111=CARTESIAN_POINT ( 'NONE',  ( -26.42409385541305511, -25.10920654474410441, 52.99999999999997158 ) ) ;
#39127=LINE ( 'NONE', #30795, #46376 ) ;
#39137=DIRECTION ( 'NONE',  ( 9.637352644315596475E-17, -0.000000000000000000, 1.000000000000000000 ) ) ;
#39138=ORIENTED_EDGE ( 'NONE', *, *, #42475, .F. ) ;
#39167=ORIENTED_EDGE ( 'NONE', *, *, #40240, .T. ) ;
#39170=AXIS2_PLACEMENT_3D ( 'NONE', #35746, #42010, #35517 ) ;
#39175=ORIENTED_EDGE ( 'NONE', *, *, #2600, .F. ) ;
#39178=DIRECTION ( 'NONE',  ( 0.000000000000000000, 1.000000000000000000, -0.000000000000000000 ) ) ;
#39215=CARTESIAN_POINT ( 'NONE',  ( -17.42409385541305511, -14.80920654474410725, 48.99999999999997868 ) ) ;
#39223=DIRECTION ( 'NONE',  ( -2.168404344971008375E-16, 0.000000000000000000, 1.000000000000000000 ) ) ;
#39233=VERTEX_POINT ( 'NONE', #32195 ) ;
#39238=( GEOMETRIC_REPRESENTATION_CONTEXT ( 3 ) GLOBAL_UNCERTAINTY_ASSIGNED_CONTEXT ( ( #10025 ) ) GLOBAL_UNIT_ASSIGNED_CONTEXT ( ( #43856, #19432, #34693 ) ) REPRESENTATION_CONTEXT ( 'NONE', 'WORKASPACE' ) );
#39254=ORIENTED_EDGE ( 'NONE', *, *, #28521, .F. ) ;
#39281=CARTESIAN_POINT ( 'NONE',  ( -6.424093855413055110, -6.859206544744110623, 47.99999999999998579 ) ) ;
#39291=VERTEX_POINT ( 'NONE', #44492 ) ;
#39292=DIRECTION ( 'NONE',  ( 1.000000000000000000, -0.000000000000000000, -0.000000000000000000 ) ) ;
#39296=CARTESIAN_POINT ( 'NONE',  ( -45.92409385541305511, -17.80920654474410370, 71.75000000000000000 ) ) ;
#39330=LINE ( 'NONE', #42307, #8526 ) ;
#39333=FACE_OUTER_BOUND ( 'NONE', #43970, .T. ) ;
#39345=EDGE_LOOP ( 'NONE', ( #18664, #3906, #25150, #34275 ) ) ;
#39351=CIRCLE ( 'NONE', #34634, 0.5000000000000004441 ) ;
#39368=EDGE_LOOP ( 'NONE', ( #10213, #7439 ) ) ;
#39378=CARTESIAN_POINT ( 'NONE',  ( -27.42409385541305511, -15.80920654474410725, 48.99999999999997868 ) ) ;
#39392=AXIS2_PLACEMENT_3D ( 'NONE', #33113, #27806, #10726 ) ;
#39402=DIRECTION ( 'NONE',  ( 0.000000000000000000, 1.000000000000000000, -0.000000000000000000 ) ) ;
#39417=AXIS2_PLACEMENT_3D ( 'NONE', #20793, #10204, #47625 ) ;
#39430=LINE ( 'NONE', #16757, #38242 ) ;
#39431=AXIS2_PLACEMENT_3D ( 'NONE', #17805, #102, #21765 ) ;
#39449=CARTESIAN_POINT ( 'NONE',  ( -8.424093855413067544, -8.109206544744111511, 50.49999999999999289 ) ) ;
#39450=ORIENTED_EDGE ( 'NONE', *, *, #14215, .F. ) ;
#39478=CARTESIAN_POINT ( 'NONE',  ( -29.92409385541305156, -6.359206544744109735, 52.99999999999997158 ) ) ;
#39488=LINE ( 'NONE', #8972, #47227 ) ;
#39497=ADVANCED_FACE ( 'NONE', ( #46080, #30351 ), #45850, .T. ) ;
#39499=ORIENTED_EDGE ( 'NONE', *, *, #15705, .T. ) ;
#39539=ORIENTED_EDGE ( 'NONE', *, *, #7324, .F. ) ;
#39558=CARTESIAN_POINT ( 'NONE',  ( -45.92409385541305511, -15.80920654474410725, 71.75000000000000000 ) ) ;
#39597=ORIENTED_EDGE ( 'NONE', *, *, #10002, .F. ) ;
#39606=ORIENTED_EDGE ( 'NONE', *, *, #38036, .F. ) ;
#39608=EDGE_CURVE ( 'NONE', #25391, #4116, #43688, .T. ) ;
#39637=LINE ( 'NONE', #27586, #36848 ) ;
#39652=FACE_OUTER_BOUND ( 'NONE', #28311, .T. ) ;
#39668=CARTESIAN_POINT ( 'NONE',  ( -20.92409385541305511, -25.10920654474410441, 81.99999999999998579 ) ) ;
#39692=CARTESIAN_POINT ( 'NONE',  ( -33.52409385541305653, -2.423472813913224222, 48.79999999999998295 ) ) ;
#39746=LINE ( 'NONE', #36283, #10354 ) ;
#39748=ORIENTED_EDGE ( 'NONE', *, *, #14520, .F. ) ;
#39793=VECTOR ( 'NONE', #31444, 1000.000000000000000 ) ;
#39811=ORIENTED_EDGE ( 'NONE', *, *, #32918, .F. ) ;
#39840=EDGE_LOOP ( 'NONE', ( #34442, #37336, #39109, #12261, #4377, #27295, #39254, #32688 ) ) ;
#39858=EDGE_CURVE ( 'NONE', #10228, #4125, #15660, .T. ) ;
#39860=DIRECTION ( 'NONE',  ( 2.081668171172170091E-15, 0.000000000000000000, -1.000000000000000000 ) ) ;
#39865=ORIENTED_EDGE ( 'NONE', *, *, #46719, .T. ) ;
#39874=CARTESIAN_POINT ( 'NONE',  ( -6.424093855413055110, -27.10920654474410796, 81.99999999999998579 ) ) ;
#39884=VERTEX_POINT ( 'NONE', #46202 ) ;
#39934=EDGE_LOOP ( 'NONE', ( #9788, #1809, #37696, #38626 ) ) ;
#39944=EDGE_CURVE ( 'NONE', #25463, #744, #28730, .T. ) ;
#39959=DIRECTION ( 'NONE',  ( -0.000000000000000000, -1.000000000000000000, -0.000000000000000000 ) ) ;
#39988=CARTESIAN_POINT ( 'NONE',  ( -27.42409385541305156, -15.80920654474410725, 47.99999999999997868 ) ) ;
#39992=CYLINDRICAL_SURFACE ( 'NONE', #48048, 0.5000000000000004441 ) ;
#40021=ORIENTED_EDGE ( 'NONE', *, *, #40454, .T. ) ;
#40036=CARTESIAN_POINT ( 'NONE',  ( -40.92409385541305511, -25.10920654474410441, 74.99999999999998579 ) ) ;
#40040=DIRECTION ( 'NONE',  ( 1.000000000000000000, -0.000000000000000000, -2.406186529621654511E-16 ) ) ;
#40047=DIRECTION ( 'NONE',  ( 0.000000000000000000, 0.000000000000000000, 1.000000000000000000 ) ) ;
#40061=CARTESIAN_POINT ( 'NONE',  ( -26.42409385541305511, -25.10920654474410441, 47.99999999999997868 ) ) ;
#40066=CARTESIAN_POINT ( 'NONE',  ( -17.42409385541305511, -14.80920654474410725, 45.99899999999998101 ) ) ;
#40120=DIRECTION ( 'NONE',  ( 0.000000000000000000, 0.000000000000000000, -1.000000000000000000 ) ) ;
#40162=DIRECTION ( 'NONE',  ( 0.000000000000000000, 0.000000000000000000, -1.000000000000000000 ) ) ;
#40165=EDGE_CURVE ( 'NONE', #28641, #11779, #8320, .T. ) ;
#40167=ORIENTED_EDGE ( 'NONE', *, *, #47728, .F. ) ;
#40191=EDGE_CURVE ( 'NONE', #29761, #11480, #31900, .T. ) ;
#40195=ORIENTED_EDGE ( 'NONE', *, *, #42083, .T. ) ;
#40212=DIRECTION ( 'NONE',  ( 0.000000000000000000, 0.000000000000000000, -1.000000000000000000 ) ) ;
#40219=ORIENTED_EDGE ( 'NONE', *, *, #5176, .F. ) ;
#40222=AXIS2_PLACEMENT_3D ( 'NONE', #22790, #39178, #37522 ) ;
#40228=EDGE_CURVE ( 'NONE', #5464, #11732, #48405, .T. ) ;
#40240=EDGE_CURVE ( 'NONE', #11393, #48283, #24839, .T. ) ;
#40301=ORIENTED_EDGE ( 'NONE', *, *, #26662, .T. ) ;
#40319=CARTESIAN_POINT ( 'NONE',  ( -8.424093855413071097, -6.359206544744109735, 52.99999999999997868 ) ) ;
#40320=DIRECTION ( 'NONE',  ( -0.000000000000000000, -0.000000000000000000, 1.000000000000000000 ) ) ;
#40338=LINE ( 'NONE', #6609, #10360 ) ;
#40352=CARTESIAN_POINT ( 'NONE',  ( -4.424093855413056886, -27.10920654474410796, 79.99999999999998579 ) ) ;
#40423=ORIENTED_EDGE ( 'NONE', *, *, #31325, .T. ) ;
#40436=AXIS2_PLACEMENT_3D ( 'NONE', #3550, #17590, #18556 ) ;
#40442=DIRECTION ( 'NONE',  ( 0.000000000000000000, 1.000000000000000000, -0.000000000000000000 ) ) ;
#40450=CARTESIAN_POINT ( 'NONE',  ( -46.92409385541305511, -17.80920654474410370, 61.49999999999999289 ) ) ;
#40454=EDGE_CURVE ( 'NONE', #3383, #28963, #18519, .T. ) ;
#40459=ORIENTED_EDGE ( 'NONE', *, *, #5890, .T. ) ;
#40469=AXIS2_PLACEMENT_3D ( 'NONE', #39281, #47158, #24269 ) ;
#40482=CARTESIAN_POINT ( 'NONE',  ( -50.42509385541305988, -8.109206544744111511, 49.44999999999998863 ) ) ;
#40484=EDGE_LOOP ( 'NONE', ( #29544, #4187 ) ) ;
#40520=LINE ( 'NONE', #29691, #33625 ) ;
#40564=AXIS2_PLACEMENT_3D ( 'NONE', #40450, #40688, #6725 ) ;
#40605=CARTESIAN_POINT ( 'NONE',  ( -27.42409385541305156, -14.65920654474411045, 52.21286476528344878 ) ) ;
#40675=CARTESIAN_POINT ( 'NONE',  ( -13.92409385541305511, -25.10920654474410441, 81.99999999999998579 ) ) ;
#40683=VERTEX_POINT ( 'NONE', #16516 ) ;
#40688=DIRECTION ( 'NONE',  ( -0.000000000000000000, 1.000000000000000000, -0.000000000000000000 ) ) ;
#40689=CARTESIAN_POINT ( 'NONE',  ( -26.42409385541305511, -6.859206544744110623, 50.50000000000000000 ) ) ;
#40695=VECTOR ( 'NONE', #33538, 1000.000000000000000 ) ;
#40699=CARTESIAN_POINT ( 'NONE',  ( -26.42409385541305511, -8.109206544744111511, 49.25000000000000000 ) ) ;
#40702=ADVANCED_FACE ( 'NONE', ( #28816 ), #17715, .T. ) ;
#40704=EDGE_CURVE ( 'NONE', #40683, #1179, #44107, .T. ) ;
#40719=DIRECTION ( 'NONE',  ( 0.1240347345892083841, 0.000000000000000000, 0.9922778767136676281 ) ) ;
#40753=DIRECTION ( 'NONE',  ( 0.000000000000000000, 0.000000000000000000, -1.000000000000000000 ) ) ;
#40768=AXIS2_PLACEMENT_3D ( 'NONE', #10421, #40442, #29119 ) ;
#40778=ORIENTED_EDGE ( 'NONE', *, *, #38718, .F. ) ;
#40785=ORIENTED_EDGE ( 'NONE', *, *, #42083, .F. ) ;
#40809=LINE ( 'NONE', #7094, #42542 ) ;
#40822=DIRECTION ( 'NONE',  ( 1.000000000000000000, -0.000000000000000000, -0.000000000000000000 ) ) ;
#40827=CARTESIAN_POINT ( 'NONE',  ( -9.424093855413055110, -25.10920654474410441, 56.99999999999997868 ) ) ;
#40828=ORIENTED_EDGE ( 'NONE', *, *, #26167, .T. ) ;
#40846=DIRECTION ( 'NONE',  ( 0.000000000000000000, -0.000000000000000000, -1.000000000000000000 ) ) ;
#40861=PLANE ( 'NONE',  #16616 ) ;
#40876=VECTOR ( 'NONE', #16195, 1000.000000000000000 ) ;
#40898=CARTESIAN_POINT ( 'NONE',  ( -6.424093855413055110, -27.10920654474410796, 47.99999999999998579 ) ) ;
#40907=AXIS2_PLACEMENT_3D ( 'NONE', #21460, #22185, #29324 ) ;
#40913=CARTESIAN_POINT ( 'NONE',  ( -28.42409385541305511, -6.859206544744110623, 47.99999999999997868 ) ) ;
#40927=AXIS2_PLACEMENT_3D ( 'NONE', #8477, #19815, #38753 ) ;
#40949=LINE ( 'NONE', #7721, #18656 ) ;
#40974=AXIS2_PLACEMENT_3D ( 'NONE', #11968, #31394, #39020 ) ;
#40985=VECTOR ( 'NONE', #29803, 1000.000000000000000 ) ;
#41002=AXIS2_PLACEMENT_3D ( 'NONE', #29548, #32521, #3204 ) ;
#41004=EDGE_CURVE ( 'NONE', #10587, #24671, #2057, .T. ) ;
#41013=ORIENTED_EDGE ( 'NONE', *, *, #42763, .T. ) ;
#41029=DIRECTION ( 'NONE',  ( 0.000000000000000000, 1.000000000000000000, -0.000000000000000000 ) ) ;
#41065=CARTESIAN_POINT ( 'NONE',  ( -27.42409385541305511, -25.10920654474410441, 63.99999999999998579 ) ) ;
#41090=CARTESIAN_POINT ( 'NONE',  ( -4.424093855413056886, -6.859206544744110623, 47.99999999999998579 ) ) ;
#41107=DIRECTION ( 'NONE',  ( -1.000000000000000000, 0.000000000000000000, 0.000000000000000000 ) ) ;
#41112=ADVANCED_FACE ( 'NONE', ( #17666 ), #28764, .F. ) ;
#41142=VECTOR ( 'NONE', #6014, 1000.000000000000000 ) ;
#41193=FACE_OUTER_BOUND ( 'NONE', #28555, .T. ) ;
#41258=CARTESIAN_POINT ( 'NONE',  ( -17.42409385541305511, -14.80920654474410725, 52.21286476528345588 ) ) ;
#41270=EDGE_LOOP ( 'NONE', ( #15789, #33606, #47841, #5856, #34895 ) ) ;
#41276=DIRECTION ( 'NONE',  ( 1.000000000000000000, -0.000000000000000000, -0.000000000000000000 ) ) ;
#41286=DIRECTION ( 'NONE',  ( 0.000000000000000000, 1.000000000000000000, -0.000000000000000000 ) ) ;
#41299=ORIENTED_EDGE ( 'NONE', *, *, #35759, .F. ) ;
#41330=LINE ( 'NONE', #37621, #24491 ) ;
#41348=ORIENTED_EDGE ( 'NONE', *, *, #41738, .F. ) ;
#41355=ADVANCED_FACE ( 'NONE', ( #41732 ), #39000, .T. ) ;
#41357=CARTESIAN_POINT ( 'NONE',  ( -7.424093855413048892, -27.10920654474410796, 63.99999999999998579 ) ) ;
#41405=DIRECTION ( 'NONE',  ( -1.000000000000000000, 0.000000000000000000, -0.000000000000000000 ) ) ;
#41413=DIRECTION ( 'NONE',  ( -0.000000000000000000, -1.000000000000000000, 0.000000000000000000 ) ) ;
#41421=FACE_OUTER_BOUND ( 'NONE', #7528, .T. ) ;
#41464=ORIENTED_EDGE ( 'NONE', *, *, #36587, .T. ) ;
#41467=CYLINDRICAL_SURFACE ( 'NONE', #15714, 0.5000000000000004441 ) ;
#41468=ADVANCED_FACE ( 'NONE', ( #24727 ), #12893, .T. ) ;
#41493=AXIS2_PLACEMENT_3D ( 'NONE', #44872, #14527, #2993 ) ;
#41516=AXIS2_PLACEMENT_3D ( 'NONE', #5233, #6196, #16780 ) ;
#41525=VERTEX_POINT ( 'NONE', #28166 ) ;
#41535=DIRECTION ( 'NONE',  ( 0.000000000000000000, 0.000000000000000000, 1.000000000000000000 ) ) ;
#41571=EDGE_LOOP ( 'NONE', ( #24535, #42806, #45433, #4114 ) ) ;
#41583=DIRECTION ( 'NONE',  ( 1.927470528863119542E-16, 0.000000000000000000, -1.000000000000000000 ) ) ;
#41590=ORIENTED_EDGE ( 'NONE', *, *, #3580, .T. ) ;
#41596=ADVANCED_FACE ( 'NONE', ( #41421 ), #29374, .F. ) ;
#41629=VECTOR ( 'NONE', #8395, 1000.000000000000000 ) ;
#41639=DIRECTION ( 'NONE',  ( -9.637352644315596475E-17, 0.000000000000000000, -1.000000000000000000 ) ) ;
#41641=CARTESIAN_POINT ( 'NONE',  ( -30.42409385541305156, -6.859206544744110623, 47.99999999999997868 ) ) ;
#41675=ADVANCED_FACE ( 'NONE', ( #37966 ), #30852, .T. ) ;
#41689=ORIENTED_EDGE ( 'NONE', *, *, #32969, .T. ) ;
#41732=FACE_OUTER_BOUND ( 'NONE', #21325, .T. ) ;
#41737=AXIS2_PLACEMENT_3D ( 'NONE', #35123, #27261, #34882 ) ;
#41738=EDGE_CURVE ( 'NONE', #733, #48469, #39430, .T. ) ;
#41745=AXIS2_PLACEMENT_3D ( 'NONE', #44772, #14194, #3140 ) ;
#41747=ORIENTED_EDGE ( 'NONE', *, *, #3947, .T. ) ;
#41748=DIRECTION ( 'NONE',  ( 0.000000000000000000, 1.000000000000000000, -0.000000000000000000 ) ) ;
#41754=EDGE_CURVE ( 'NONE', #20983, #42591, #6790, .T. ) ;
#41756=ORIENTED_EDGE ( 'NONE', *, *, #18650, .T. ) ;
#41762=VERTEX_POINT ( 'NONE', #13061 ) ;
#41765=PLANE ( 'NONE',  #20766 ) ;
#41772=CYLINDRICAL_SURFACE ( 'NONE', #39170, 1.999999999999994893 ) ;
#41785=CARTESIAN_POINT ( 'NONE',  ( -6.424093855413055110, -6.859206544744110623, 45.99999999999998579 ) ) ;
#41792=CARTESIAN_POINT ( 'NONE',  ( -6.424093855413058662, -6.359206544744109735, 52.99999999999998579 ) ) ;
#41832=VECTOR ( 'NONE', #22684, 1000.000000000000000 ) ;
#41859=DIRECTION ( 'NONE',  ( -1.000000000000000000, 0.000000000000000000, 0.000000000000000000 ) ) ;
#41861=EDGE_CURVE ( 'NONE', #11264, #27788, #37463, .T. ) ;
#41877=EDGE_CURVE ( 'NONE', #31526, #5342, #29307, .T. ) ;
#41878=ORIENTED_EDGE ( 'NONE', *, *, #36980, .T. ) ;
#41887=CARTESIAN_POINT ( 'NONE',  ( -15.92409385541305333, -14.80920654474410547, 48.99999999999997868 ) ) ;
#41888=ORIENTED_EDGE ( 'NONE', *, *, #13703, .F. ) ;
#41913=ORIENTED_EDGE ( 'NONE', *, *, #4931, .F. ) ;
#41916=ORIENTED_EDGE ( 'NONE', *, *, #2306, .F. ) ;
#41929=VERTEX_POINT ( 'NONE', #42343 ) ;
#41954=FACE_BOUND ( 'NONE', #48670, .T. ) ;
#41970=DIRECTION ( 'NONE',  ( 0.000000000000000000, 0.000000000000000000, -1.000000000000000000 ) ) ;
#41984=EDGE_CURVE ( 'NONE', #31166, #45033, #25668, .T. ) ;
#41987=VERTEX_POINT ( 'NONE', #30789 ) ;
#42010=DIRECTION ( 'NONE',  ( -0.000000000000000000, -1.000000000000000000, -0.000000000000000000 ) ) ;
#42012=EDGE_LOOP ( 'NONE', ( #17977, #28004, #35402, #28048, #38075 ) ) ;
#42034=VECTOR ( 'NONE', #32791, 1000.000000000000114 ) ;
#42042=DIRECTION ( 'NONE',  ( 2.181982678098338148E-16, 0.000000000000000000, -1.000000000000000000 ) ) ;
#42052=LINE ( 'NONE', #31206, #1373 ) ;
#42054=CARTESIAN_POINT ( 'NONE',  ( -6.424093855413055110, -6.859206544744110623, 47.99999999999998579 ) ) ;
#42083=EDGE_CURVE ( 'NONE', #12097, #13748, #13869, .T. ) ;
#42103=CARTESIAN_POINT ( 'NONE',  ( -9.424093855413055110, -25.10920654474410441, 54.99999999999997868 ) ) ;
#42106=FACE_OUTER_BOUND ( 'NONE', #26557, .T. ) ;
#42108=ORIENTED_EDGE ( 'NONE', *, *, #41738, .T. ) ;
#42114=VERTEX_POINT ( 'NONE', #20166 ) ;
#42131=DIRECTION ( 'NONE',  ( 0.000000000000000000, 0.000000000000000000, -1.000000000000000000 ) ) ;
#42182=DIRECTION ( 'NONE',  ( 0.000000000000000000, 1.000000000000000000, -0.000000000000000000 ) ) ;
#42213=CARTESIAN_POINT ( 'NONE',  ( -13.92409385541305511, -10.60920654474410618, 81.49999999999998579 ) ) ;
#42237=ORIENTED_EDGE ( 'NONE', *, *, #41004, .F. ) ;
#42254=FACE_OUTER_BOUND ( 'NONE', #17938, .T. ) ;
#42262=DIRECTION ( 'NONE',  ( 1.927470528863119542E-16, 0.000000000000000000, -1.000000000000000000 ) ) ;
#42306=ORIENTED_EDGE ( 'NONE', *, *, #13351, .F. ) ;
#42307=CARTESIAN_POINT ( 'NONE',  ( -33.52409385541305653, -8.109206544744111511, 49.44999999999998863 ) ) ;
#42320=DIRECTION ( 'NONE',  ( 0.000000000000000000, -0.000000000000000000, -1.000000000000000000 ) ) ;
#42343=CARTESIAN_POINT ( 'NONE',  ( -28.42409385541305511, -6.859206544744110623, 45.99999999999998579 ) ) ;
#42347=CIRCLE ( 'NONE', #35261, 0.5000000000000004441 ) ;
#42363=ORIENTED_EDGE ( 'NONE', *, *, #44150, .T. ) ;
#42382=EDGE_LOOP ( 'NONE', ( #46141, #8605, #28804, #14612 ) ) ;
#42410=VECTOR ( 'NONE', #21157, 1000.000000000000000 ) ;
#42423=VERTEX_POINT ( 'NONE', #19633 ) ;
#42451=ORIENTED_EDGE ( 'NONE', *, *, #45204, .F. ) ;
#42453=CIRCLE ( 'NONE', #22801, 1.000000000000000888 ) ;
#42473=DIRECTION ( 'NONE',  ( -1.000000000000000000, 0.000000000000000000, 0.000000000000000000 ) ) ;
#42475=EDGE_CURVE ( 'NONE', #41987, #31278, #19383, .T. ) ;
#42484=ORIENTED_EDGE ( 'NONE', *, *, #37500, .T. ) ;
#42515=LINE ( 'NONE', #24284, #2906 ) ;
#42538=ORIENTED_EDGE ( 'NONE', *, *, #14022, .T. ) ;
#42542=VECTOR ( 'NONE', #17896, 1000.000000000000000 ) ;
#42554=CIRCLE ( 'NONE', #41737, 2.000000000000001776 ) ;
#42591=VERTEX_POINT ( 'NONE', #15345 ) ;
#42628=DIRECTION ( 'NONE',  ( 0.000000000000000000, 0.000000000000000000, 1.000000000000000000 ) ) ;
#42644=DIRECTION ( 'NONE',  ( -0.000000000000000000, -1.000000000000000000, -0.000000000000000000 ) ) ;
#42661=CARTESIAN_POINT ( 'NONE',  ( -20.92409385541305511, -10.10920654474410618, 80.49999999999998579 ) ) ;
#42671=FACE_OUTER_BOUND ( 'NONE', #36167, .T. ) ;
#42682=DIRECTION ( 'NONE',  ( -0.000000000000000000, -1.000000000000000000, 0.000000000000000000 ) ) ;
#42687=ORIENTED_EDGE ( 'NONE', *, *, #36374, .T. ) ;
#42688=DIRECTION ( 'NONE',  ( 0.000000000000000000, 0.000000000000000000, 1.000000000000000000 ) ) ;
#42708=CARTESIAN_POINT ( 'NONE',  ( -33.52409385541305653, -6.359206544744109735, 49.44999999999998863 ) ) ;
#42725=VERTEX_POINT ( 'NONE', #24943 ) ;
#42741=AXIS2_PLACEMENT_3D ( 'NONE', #2855, #22310, #17862 ) ;
#42742=CARTESIAN_POINT ( 'NONE',  ( -50.42509385541305988, -8.109206544744111511, 50.49999999999998579 ) ) ;
#42761=EDGE_LOOP ( 'NONE', ( #34174, #3289, #14748, #43770 ) ) ;
#42763=EDGE_CURVE ( 'NONE', #32365, #733, #37497, .T. ) ;
#42770=ORIENTED_EDGE ( 'NONE', *, *, #33839, .T. ) ;
#42772=DIRECTION ( 'NONE',  ( -1.000000000000000000, -0.000000000000000000, -0.000000000000000000 ) ) ;
#42806=ORIENTED_EDGE ( 'NONE', *, *, #13746, .F. ) ;
#42813=LINE ( 'NONE', #12279, #40876 ) ;
#42822=ADVANCED_FACE ( 'NONE', ( #42106 ), #23155, .F. ) ;
#42862=ORIENTED_EDGE ( 'NONE', *, *, #46719, .F. ) ;
#42868=DIRECTION ( 'NONE',  ( 1.000000000000000000, 0.000000000000000000, 0.000000000000000000 ) ) ;
#42892=EDGE_CURVE ( 'NONE', #44110, #115, #10969, .T. ) ;
#42931=DIRECTION ( 'NONE',  ( 0.000000000000000000, 0.000000000000000000, 1.000000000000000000 ) ) ;
#42933=ORIENTED_EDGE ( 'NONE', *, *, #1713, .T. ) ;
#42939=ORIENTED_EDGE ( 'NONE', *, *, #374, .F. ) ;
#42946=EDGE_CURVE ( 'NONE', #5216, #37238, #39093, .T. ) ;
#42975=EDGE_CURVE ( 'NONE', #37066, #23568, #1331, .T. ) ;
#43005=AXIS2_PLACEMENT_3D ( 'NONE', #19084, #41748, #30432 ) ;
#43029=VERTEX_POINT ( 'NONE', #26964 ) ;
#43031=UNCERTAINTY_MEASURE_WITH_UNIT (LENGTH_MEASURE( 1.000000000000000082E-05 ), #15533, 'distance_accuracy_value', 'NONE');
#43043=CARTESIAN_POINT ( 'NONE',  ( -35.32409385541306079, -25.10920654474410441, 52.29999999999998295 ) ) ;
#43055=CYLINDRICAL_SURFACE ( 'NONE', #28398, 1.999999999999994893 ) ;
#43069=CARTESIAN_POINT ( 'NONE',  ( -33.95962776134579286, -8.109206544744111511, 50.50000000000000000 ) ) ;
#43092=DIRECTION ( 'NONE',  ( 0.000000000000000000, 0.000000000000000000, 1.000000000000000000 ) ) ;
#43100=CIRCLE ( 'NONE', #28930, 1.999999999999994893 ) ;
#43180=ORIENTED_EDGE ( 'NONE', *, *, #41861, .F. ) ;
#43201=EDGE_LOOP ( 'NONE', ( #6061, #7562 ) ) ;
#43206=FACE_OUTER_BOUND ( 'NONE', #18190, .T. ) ;
#43211=LINE ( 'NONE', #27699, #41142 ) ;
#43246=DIRECTION ( 'NONE',  ( 1.927470528863119542E-16, 0.000000000000000000, -1.000000000000000000 ) ) ;
#43249=EDGE_CURVE ( 'NONE', #27864, #12986, #29644, .T. ) ;
#43250=ADVANCED_FACE ( 'NONE', ( #36029 ), #2310, .F. ) ;
#43266=DIRECTION ( 'NONE',  ( -0.000000000000000000, -1.000000000000000000, -0.000000000000000000 ) ) ;
#43283=AXIS2_PLACEMENT_3D ( 'NONE', #44847, #26123, #31513 ) ;
#43306=CARTESIAN_POINT ( 'NONE',  ( -8.424093855413053333, -15.80920654474410725, 47.99999999999998579 ) ) ;
#43334=CARTESIAN_POINT ( 'NONE',  ( -20.92409385541305511, -10.60920654474410618, 81.99999999999998579 ) ) ;
#43346=ADVANCED_FACE ( 'NONE', ( #41193 ), #45383, .F. ) ;
#43381=EDGE_CURVE ( 'NONE', #2631, #12097, #40949, .T. ) ;
#43389=CARTESIAN_POINT ( 'NONE',  ( -35.32409385541306079, -8.109206544744111511, 51.54999999999998295 ) ) ;
#43394=ORIENTED_EDGE ( 'NONE', *, *, #43585, .T. ) ;
#43409=VERTEX_POINT ( 'NONE', #33531 ) ;
#43441=DIRECTION ( 'NONE',  ( 0.000000000000000000, 0.000000000000000000, -1.000000000000000000 ) ) ;
#43465=CARTESIAN_POINT ( 'NONE',  ( -13.92409385541305511, -10.10920654474410618, 81.49999999999998579 ) ) ;
#43536=LINE ( 'NONE', #2399, #350 ) ;
#43548=DIRECTION ( 'NONE',  ( 0.000000000000000000, 0.000000000000000000, -1.000000000000000000 ) ) ;
#43563=CARTESIAN_POINT ( 'NONE',  ( -17.42409385541305511, -14.80920654474410725, 47.99999999999998579 ) ) ;
#43570=EDGE_CURVE ( 'NONE', #31120, #1645, #44589, .T. ) ;
#43585=EDGE_CURVE ( 'NONE', #7661, #48493, #4510, .T. ) ;
#43588=CARTESIAN_POINT ( 'NONE',  ( -27.42409385541305511, -10.10920654474410618, 79.49999999999998579 ) ) ;
#43605=DIRECTION ( 'NONE',  ( -0.000000000000000000, 0.000000000000000000, 1.000000000000000000 ) ) ;
#43643=DIRECTION ( 'NONE',  ( 1.000000000000000000, 0.000000000000000000, -0.000000000000000000 ) ) ;
#43645=CARTESIAN_POINT ( 'NONE',  ( -4.424093855413056886, -27.10920654474410796, 47.99999999999998579 ) ) ;
#43666=CARTESIAN_POINT ( 'NONE',  ( -6.424093855413058662, -25.10920654474410441, 52.99999999999998579 ) ) ;
#43681=EDGE_LOOP ( 'NONE', ( #2712, #37256, #22134, #41916 ) ) ;
#43688=CIRCLE ( 'NONE', #25561, 1.250000000000007994 ) ;
#43700=LINE ( 'NONE', #16600, #25763 ) ;
#43746=LINE ( 'NONE', #47668, #12318 ) ;
#43770=ORIENTED_EDGE ( 'NONE', *, *, #24938, .F. ) ;
#43796=DIRECTION ( 'NONE',  ( 0.000000000000000000, 0.000000000000000000, 1.000000000000000000 ) ) ;
#43799=CARTESIAN_POINT ( 'NONE',  ( -4.924093855413050669, -6.359206544744109735, 52.99999999999998579 ) ) ;
#43808=VERTEX_POINT ( 'NONE', #2671 ) ;
#43827=CARTESIAN_POINT ( 'NONE',  ( -4.424093855413049781, -6.859206544744110623, 52.99999999999998579 ) ) ;
#43856=( LENGTH_UNIT ( ) NAMED_UNIT ( * ) SI_UNIT ( .MILLI., .METRE. ) );
#43857=DIRECTION ( 'NONE',  ( 1.000000000000000000, -0.000000000000000000, -8.260587980841940012E-17 ) ) ;
#43861=AXIS2_PLACEMENT_3D ( 'NONE', #22182, #10844, #11832 ) ;
#43882=DIRECTION ( 'NONE',  ( 1.000000000000000000, 0.000000000000000000, -5.466375705775733989E-17 ) ) ;
#43887=APPLICATION_CONTEXT ( 'automotive_design' ) ;
#43891=DIRECTION ( 'NONE',  ( 0.000000000000000000, 1.000000000000000000, -0.000000000000000000 ) ) ;
#43942=AXIS2_PLACEMENT_3D ( 'NONE', #26294, #451, #23101 ) ;
#43953=LINE ( 'NONE', #44203, #32831 ) ;
#43958=CARTESIAN_POINT ( 'NONE',  ( -28.42409385541305511, -25.10920654474410441, 54.99999999999996447 ) ) ;
#43970=EDGE_LOOP ( 'NONE', ( #10348, #13922, #43180, #7551, #5182, #35119, #20063, #31395, #7592, #31835 ) ) ;
#43972=AXIS2_PLACEMENT_3D ( 'NONE', #16241, #39402, #8892 ) ;
#43974=ORIENTED_EDGE ( 'NONE', *, *, #41984, .F. ) ;
#44000=AXIS2_PLACEMENT_3D ( 'NONE', #20944, #35944, #2221 ) ;
#44007=AXIS2_PLACEMENT_3D ( 'NONE', #20026, #37998, #42688 ) ;
#44030=CARTESIAN_POINT ( 'NONE',  ( -7.424093855413048892, -25.10920654474410441, 56.99999999999997868 ) ) ;
#44053=DIRECTION ( 'NONE',  ( 1.000000000000000000, 0.000000000000000000, 0.000000000000000000 ) ) ;
#44063=VERTEX_POINT ( 'NONE', #30500 ) ;
#44070=ORIENTED_EDGE ( 'NONE', *, *, #37544, .F. ) ;
#44075=LINE ( 'NONE', #13508, #14725 ) ;
#44083=AXIS2_PLACEMENT_3D ( 'NONE', #36071, #17597, #29665 ) ;
#44101=DIRECTION ( 'NONE',  ( 0.000000000000000000, -1.000000000000000000, 0.000000000000000000 ) ) ;
#44102=ORIENTED_EDGE ( 'NONE', *, *, #2376, .T. ) ;
#44107=LINE ( 'NONE', #10825, #3590 ) ;
#44110=VERTEX_POINT ( 'NONE', #5112 ) ;
#44144=ORIENTED_EDGE ( 'NONE', *, *, #45880, .T. ) ;
#44150=EDGE_CURVE ( 'NONE', #44500, #48597, #42052, .T. ) ;
#44203=CARTESIAN_POINT ( 'NONE',  ( -48.42409385541304800, -25.10920654474410441, 81.99999999999998579 ) ) ;
#44207=CARTESIAN_POINT ( 'NONE',  ( -35.32409385541306079, -6.359206544744109735, 48.79999999999998295 ) ) ;
#44220=DIRECTION ( 'NONE',  ( 0.000000000000000000, 0.000000000000000000, 1.000000000000000000 ) ) ;
#44260=CARTESIAN_POINT ( 'NONE',  ( -9.424093855413051557, -25.10920654474410441, 78.99999999999998579 ) ) ;
#44279=LINE ( 'NONE', #36369, #31064 ) ;
#44353=ORIENTED_EDGE ( 'NONE', *, *, #23395, .T. ) ;
#44354=DIRECTION ( 'NONE',  ( 2.775557561562888984E-15, 0.000000000000000000, -1.000000000000000000 ) ) ;
#44357=VERTEX_POINT ( 'NONE', #48394 ) ;
#44358=CARTESIAN_POINT ( 'NONE',  ( -28.42409385541305511, -25.10920654474410441, 47.99999999999997868 ) ) ;
#44375=EDGE_CURVE ( 'NONE', #45181, #20101, #25508, .T. ) ;
#44435=CARTESIAN_POINT ( 'NONE',  ( -4.424093855413056886, -8.109206544744111511, 49.24999999999999289 ) ) ;
#44439=ORIENTED_EDGE ( 'NONE', *, *, #31630, .T. ) ;
#44442=CARTESIAN_POINT ( 'NONE',  ( -19.92409385541305511, -14.80920654474410725, 45.99899999999998101 ) ) ;
#44445=ORIENTED_EDGE ( 'NONE', *, *, #29800, .T. ) ;
#44448=EDGE_LOOP ( 'NONE', ( #24636, #5276, #11033, #39138, #34319 ) ) ;
#44457=EDGE_CURVE ( 'NONE', #45033, #42114, #40520, .T. ) ;
#44470=CARTESIAN_POINT ( 'NONE',  ( -18.92409385541305511, -15.80920654474410725, 47.99999999999997868 ) ) ;
#44487=ORIENTED_EDGE ( 'NONE', *, *, #29042, .F. ) ;
#44492=CARTESIAN_POINT ( 'NONE',  ( -50.42409385541304800, -25.10920654474410441, 79.99999999999998579 ) ) ;
#44500=VERTEX_POINT ( 'NONE', #45453 ) ;
#44505=DIRECTION ( 'NONE',  ( 1.000000000000000000, 0.000000000000000000, 1.927470528863119295E-16 ) ) ;
#44530=ADVANCED_FACE ( 'NONE', ( #31579 ), #5959, .T. ) ;
#44563=FACE_OUTER_BOUND ( 'NONE', #33392, .T. ) ;
#44568=DIRECTION ( 'NONE',  ( 0.000000000000000000, 0.000000000000000000, 1.000000000000000000 ) ) ;
#44589=LINE ( 'NONE', #37164, #15486 ) ;
#44617=LINE ( 'NONE', #29842, #20420 ) ;
#44639=FACE_OUTER_BOUND ( 'NONE', #46113, .T. ) ;
#44650=ORIENTED_EDGE ( 'NONE', *, *, #48088, .T. ) ;
#44727=MECHANICAL_DESIGN_GEOMETRIC_PRESENTATION_REPRESENTATION('',(#3018),#2247);
#44747=VECTOR ( 'NONE', #25946, 1000.000000000000000 ) ;
#44767=ORIENTED_EDGE ( 'NONE', *, *, #5176, .T. ) ;
#44772=CARTESIAN_POINT ( 'NONE',  ( -28.42409385541305511, -25.10920654474410441, 47.99999999999997868 ) ) ;
#44783=ORIENTED_EDGE ( 'NONE', *, *, #14831, .F. ) ;
#44811=EDGE_LOOP ( 'NONE', ( #30381, #33786, #23812, #12368 ) ) ;
#44830=DIRECTION ( 'NONE',  ( -1.000000000000000000, 0.000000000000000000, 3.652049423109068320E-16 ) ) ;
#44837=AXIS2_PLACEMENT_3D ( 'NONE', #19129, #48428, #22843 ) ;
#44842=VECTOR ( 'NONE', #39860, 1000.000000000000000 ) ;
#44847=CARTESIAN_POINT ( 'NONE',  ( -28.42409385541305511, -6.359206544744109735, 52.99999999999997158 ) ) ;
#44857=CARTESIAN_POINT ( 'NONE',  ( -35.32409385541306079, -6.359206544744109735, 52.29999999999998295 ) ) ;
#44872=CARTESIAN_POINT ( 'NONE',  ( -6.424093855413055110, -25.10920654474410441, 47.99999999999998579 ) ) ;
#44890=AXIS2_PLACEMENT_3D ( 'NONE', #35774, #27677, #20044 ) ;
#44896=CYLINDRICAL_SURFACE ( 'NONE', #23697, 1.250000000000001110 ) ;
#44900=ORIENTED_EDGE ( 'NONE', *, *, #23477, .F. ) ;
#44928=DIRECTION ( 'NONE',  ( -1.000000000000000000, 0.000000000000000000, 0.000000000000000000 ) ) ;
#44954=VECTOR ( 'NONE', #17123, 1000.000000000000000 ) ;
#44964=EDGE_LOOP ( 'NONE', ( #26103, #27823, #1860, #26144, #28075, #22313, #35795, #41689, #15514, #46623, #41299, #33082, #29346, #1148 ) ) ;
#44972=PLANE ( 'NONE',  #43005 ) ;
#45033=VERTEX_POINT ( 'NONE', #43827 ) ;
#45046=VERTEX_POINT ( 'NONE', #17204 ) ;
#45049=ORIENTED_EDGE ( 'NONE', *, *, #36374, .F. ) ;
#45054=ORIENTED_EDGE ( 'NONE', *, *, #43570, .F. ) ;
#45084=EDGE_LOOP ( 'NONE', ( #2314, #7740, #19443, #22401, #44650, #39010 ) ) ;
#45108=EDGE_LOOP ( 'NONE', ( #46950, #33893, #9783, #42538 ) ) ;
#45157=DIRECTION ( 'NONE',  ( 0.000000000000000000, 1.000000000000000000, -0.000000000000000000 ) ) ;
#45158=ORIENTED_EDGE ( 'NONE', *, *, #18900, .T. ) ;
#45171=DIRECTION ( 'NONE',  ( -0.000000000000000000, 1.000000000000000000, -0.000000000000000000 ) ) ;
#45175=CARTESIAN_POINT ( 'NONE',  ( -45.92409385541305511, -17.80920654474410370, 69.24999999999998579 ) ) ;
#45181=VERTEX_POINT ( 'NONE', #14696 ) ;
#45204=EDGE_CURVE ( 'NONE', #20983, #30760, #652, .T. ) ;
#45222=FACE_OUTER_BOUND ( 'NONE', #39934, .T. ) ;
#45240=EDGE_CURVE ( 'NONE', #11480, #30462, #39330, .T. ) ;
#45246=EDGE_CURVE ( 'NONE', #2100, #48493, #27998, .T. ) ;
#45284=ORIENTED_EDGE ( 'NONE', *, *, #2535, .F. ) ;
#45333=PLANE ( 'NONE',  #17941 ) ;
#45345=DIRECTION ( 'NONE',  ( 2.181982678098338148E-16, 0.000000000000000000, -1.000000000000000000 ) ) ;
#45380=CARTESIAN_POINT ( 'NONE',  ( -40.92409385541305511, -15.80920654474410725, 74.99999999999998579 ) ) ;
#45383=CYLINDRICAL_SURFACE ( 'NONE', #14691, 1.250000000000001110 ) ;
#45403=AXIS2_PLACEMENT_3D ( 'NONE', #381, #11698, #19323 ) ;
#45414=VECTOR ( 'NONE', #6258, 1000.000000000000000 ) ;
#45418=VERTEX_POINT ( 'NONE', #40061 ) ;
#45431=DIRECTION ( 'NONE',  ( 0.000000000000000000, 0.000000000000000000, 1.000000000000000000 ) ) ;
#45433=ORIENTED_EDGE ( 'NONE', *, *, #21881, .F. ) ;
#45453=CARTESIAN_POINT ( 'NONE',  ( -50.42409385541304800, -27.10920654474410796, 47.99999999999998579 ) ) ;
#45492=LINE ( 'NONE', #28469, #22053 ) ;
#45506=CARTESIAN_POINT ( 'NONE',  ( -16.92409385541305511, -14.80920654474410547, 52.21286476528345588 ) ) ;
#45512=FACE_OUTER_BOUND ( 'NONE', #45542, .T. ) ;
#45542=EDGE_LOOP ( 'NONE', ( #47193, #32092, #33933, #8519 ) ) ;
#45573=ADVANCED_FACE ( 'NONE', ( #26983 ), #35084, .T. ) ;
#45581=DIRECTION ( 'NONE',  ( -0.000000000000000000, 0.000000000000000000, 1.000000000000000000 ) ) ;
#45583=ORIENTED_EDGE ( 'NONE', *, *, #18831, .T. ) ;
#45632=AXIS2_PLACEMENT_3D ( 'NONE', #40827, #37608, #4154 ) ;
#45646=EDGE_CURVE ( 'NONE', #12097, #25463, #12688, .T. ) ;
#45656=PLANE ( 'NONE',  #30018 ) ;
#45667=DIRECTION ( 'NONE',  ( -1.000000000000000000, 0.000000000000000000, 0.000000000000000000 ) ) ;
#45770=CARTESIAN_POINT ( 'NONE',  ( -17.02409385541305653, -14.80920654474410725, 47.99999999999998579 ) ) ;
#45798=ORIENTED_EDGE ( 'NONE', *, *, #37544, .T. ) ;
#45810=EDGE_LOOP ( 'NONE', ( #48362, #35054, #20976, #8047, #19124 ) ) ;
#45812=CARTESIAN_POINT ( 'NONE',  ( -27.42409385541305511, -25.10920654474410441, 54.99999999999997868 ) ) ;
#45818=CYLINDRICAL_SURFACE ( 'NONE', #43283, 1.999999999999994893 ) ;
#45850=PLANE ( 'NONE',  #9059 ) ;
#45855=SURFACE_STYLE_USAGE ( .BOTH. , #4242 ) ;
#45861=ORIENTED_EDGE ( 'NONE', *, *, #25640, .F. ) ;
#45871=ORIENTED_EDGE ( 'NONE', *, *, #33839, .F. ) ;
#45880=EDGE_CURVE ( 'NONE', #21727, #40683, #17976, .T. ) ;
#45886=DIRECTION ( 'NONE',  ( 1.000000000000000000, 0.000000000000000000, 0.000000000000000000 ) ) ;
#45896=ORIENTED_EDGE ( 'NONE', *, *, #18900, .F. ) ;
#45914=ORIENTED_EDGE ( 'NONE', *, *, #35322, .T. ) ;
#45927=VECTOR ( 'NONE', #30943, 1000.000000000000000 ) ;
#45992=FACE_OUTER_BOUND ( 'NONE', #4449, .T. ) ;
#45993=DIRECTION ( 'NONE',  ( 0.000000000000000000, 1.000000000000000000, -0.000000000000000000 ) ) ;
#45997=ORIENTED_EDGE ( 'NONE', *, *, #28242, .T. ) ;
#46019=DIRECTION ( 'NONE',  ( -8.260587980841940012E-17, 0.000000000000000000, -1.000000000000000000 ) ) ;
#46064=AXIS2_PLACEMENT_3D ( 'NONE', #46144, #38503, #34311 ) ;
#46080=FACE_BOUND ( 'NONE', #39368, .T. ) ;
#46090=ORIENTED_EDGE ( 'NONE', *, *, #44457, .T. ) ;
#46113=EDGE_LOOP ( 'NONE', ( #10733, #7411, #47320, #23445, #12833, #39167 ) ) ;
#46130=LINE ( 'NONE', #27899, #37856 ) ;
#46133=DIRECTION ( 'NONE',  ( -0.000000000000000000, -1.000000000000000000, 0.000000000000000000 ) ) ;
#46141=ORIENTED_EDGE ( 'NONE', *, *, #24957, .F. ) ;
#46143=VECTOR ( 'NONE', #17850, 1000.000000000000000 ) ;
#46144=CARTESIAN_POINT ( 'NONE',  ( -17.42409385541305511, -14.80920654474410725, 48.99999999999997868 ) ) ;
#46174=EDGE_CURVE ( 'NONE', #43409, #36016, #15574, .T. ) ;
#46184=DIRECTION ( 'NONE',  ( 0.9922778767136677391, 0.000000000000000000, -0.1240347345892083841 ) ) ;
#46202=CARTESIAN_POINT ( 'NONE',  ( -48.42409385541304800, -25.10920654474410441, 45.99999999999998579 ) ) ;
#46211=CARTESIAN_POINT ( 'NONE',  ( -29.92409385541305156, -6.359206544744109735, 52.99999999999997158 ) ) ;
#46219=CARTESIAN_POINT ( 'NONE',  ( -30.42409385541305156, -8.109206544744111511, 50.50000000000000000 ) ) ;
#46256=ORIENTED_EDGE ( 'NONE', *, *, #6613, .T. ) ;
#46265=DIRECTION ( 'NONE',  ( -1.000000000000000000, 0.000000000000000000, -0.000000000000000000 ) ) ;
#46286=AXIS2_PLACEMENT_3D ( 'NONE', #28246, #9781, #47924 ) ;
#46305=CIRCLE ( 'NONE', #3046, 1.000000000000000888 ) ;
#46327=CARTESIAN_POINT ( 'NONE',  ( -9.424093855413051557, -25.10920654474410441, 77.00000000000000000 ) ) ;
#46331=ORIENTED_EDGE ( 'NONE', *, *, #37709, .T. ) ;
#46362=PLANE ( 'NONE',  #5802 ) ;
#46367=CARTESIAN_POINT ( 'NONE',  ( -35.32409385541306079, -2.423472813913224222, 48.79999999999998295 ) ) ;
#46376=VECTOR ( 'NONE', #5167, 1000.000000000000000 ) ;
#46381=LINE ( 'NONE', #35278, #22765 ) ;
#46417=CARTESIAN_POINT ( 'NONE',  ( -27.42409385541305511, -15.80920654474410725, 63.99999999999998579 ) ) ;
#46471=DIRECTION ( 'NONE',  ( -1.000000000000000000, 0.000000000000000000, 0.000000000000000000 ) ) ;
#46489=VECTOR ( 'NONE', #31342, 1000.000000000000000 ) ;
#46495=DIRECTION ( 'NONE',  ( 0.000000000000000000, 1.000000000000000000, 0.000000000000000000 ) ) ;
#46498=DIRECTION ( 'NONE',  ( 0.000000000000000000, 0.000000000000000000, 1.000000000000000000 ) ) ;
#46505=DIRECTION ( 'NONE',  ( 0.000000000000000000, 0.000000000000000000, 1.000000000000000000 ) ) ;
#46513=SHAPE_REPRESENTATION ( 'Base Cast Iron Chassis Plate', ( #29031 ), #39238 ) ;
#46538=VECTOR ( 'NONE', #7524, 1000.000000000000000 ) ;
#46549=CARTESIAN_POINT ( 'NONE',  ( -18.92409385541305511, -15.80920654474410725, 48.99999999999997868 ) ) ;
#46566=CARTESIAN_POINT ( 'NONE',  ( -35.32409385541306079, -25.10920654474410441, 52.29999999999998295 ) ) ;
#46589=EDGE_CURVE ( 'NONE', #30760, #37238, #7681, .T. ) ;
#46602=ORIENTED_EDGE ( 'NONE', *, *, #40191, .T. ) ;
#46623=ORIENTED_EDGE ( 'NONE', *, *, #6962, .T. ) ;
#46625=DIRECTION ( 'NONE',  ( 0.000000000000000000, 0.000000000000000000, 1.000000000000000000 ) ) ;
#46631=CARTESIAN_POINT ( 'NONE',  ( -17.42409385541305511, -14.80920654474410725, 52.21286476528345588 ) ) ;
#46651=ADVANCED_FACE ( 'NONE', ( #23669 ), #1967, .T. ) ;
#46657=EDGE_CURVE ( 'NONE', #23568, #37066, #5472, .T. ) ;
#46659=CARTESIAN_POINT ( 'NONE',  ( -17.92409385541305511, -14.80920654474410547, 48.99999999999997868 ) ) ;
#46719=EDGE_CURVE ( 'NONE', #31278, #36791, #9126, .T. ) ;
#46767=ORIENTED_EDGE ( 'NONE', *, *, #45880, .F. ) ;
#46770=CARTESIAN_POINT ( 'NONE',  ( -4.424093855413056886, -6.859206544744110623, 50.49999999999999289 ) ) ;
#46791=ORIENTED_EDGE ( 'NONE', *, *, #35717, .F. ) ;
#46817=ORIENTED_EDGE ( 'NONE', *, *, #16023, .T. ) ;
#46863=DIRECTION ( 'NONE',  ( 0.000000000000000000, 1.000000000000000000, -0.000000000000000000 ) ) ;
#46864=DIRECTION ( 'NONE',  ( -1.000000000000000000, 0.000000000000000000, 0.000000000000000000 ) ) ;
#46884=LINE ( 'NONE', #9943, #15151 ) ;
#46885=ORIENTED_EDGE ( 'NONE', *, *, #47728, .T. ) ;
#46888=EDGE_CURVE ( 'NONE', #48469, #24724, #16123, .T. ) ;
#46913=ORIENTED_EDGE ( 'NONE', *, *, #6379, .F. ) ;
#46918=VERTEX_POINT ( 'NONE', #34123 ) ;
#46922=ORIENTED_EDGE ( 'NONE', *, *, #25100, .F. ) ;
#46940=VECTOR ( 'NONE', #10285, 1000.000000000000000 ) ;
#46943=FACE_OUTER_BOUND ( 'NONE', #41270, .T. ) ;
#46950=ORIENTED_EDGE ( 'NONE', *, *, #18691, .F. ) ;
#46968=AXIS2_PLACEMENT_3D ( 'NONE', #31667, #8532, #15657 ) ;
#46969=EDGE_CURVE ( 'NONE', #38652, #36016, #31660, .T. ) ;
#47002=VECTOR ( 'NONE', #4664, 1000.000000000000000 ) ;
#47025=CARTESIAN_POINT ( 'NONE',  ( -45.92409385541305511, -15.80920654474410725, 70.50000000000000000 ) ) ;
#47029=CARTESIAN_POINT ( 'NONE',  ( -42.07024770156689897, -15.80920654474410725, 65.83076923076922071 ) ) ;
#47044=FACE_OUTER_BOUND ( 'NONE', #19407, .T. ) ;
#47058=ORIENTED_EDGE ( 'NONE', *, *, #30697, .T. ) ;
#47087=CIRCLE ( 'NONE', #32155, 1.250000000000001110 ) ;
#47094=DIRECTION ( 'NONE',  ( 1.000000000000000000, -6.938893903907222067E-14, 0.000000000000000000 ) ) ;
#47097=DIRECTION ( 'NONE',  ( -0.000000000000000000, -1.000000000000000000, -0.000000000000000000 ) ) ;
#47148=VECTOR ( 'NONE', #15159, 1000.000000000000000 ) ;
#47158=DIRECTION ( 'NONE',  ( -0.000000000000000000, -1.000000000000000000, 0.000000000000000000 ) ) ;
#47171=CARTESIAN_POINT ( 'NONE',  ( -17.42409385541305511, -14.80920654474410725, 47.99999999999998579 ) ) ;
#47193=ORIENTED_EDGE ( 'NONE', *, *, #9948, .F. ) ;
#47219=VERTEX_POINT ( 'NONE', #8235 ) ;
#47227=VECTOR ( 'NONE', #4788, 1000.000000000000000 ) ;
#47239=AXIS2_PLACEMENT_3D ( 'NONE', #25422, #11549, #37637 ) ;
#47241=FACE_OUTER_BOUND ( 'NONE', #47957, .T. ) ;
#47259=LINE ( 'NONE', #39378, #42410 ) ;
#47292=ORIENTED_EDGE ( 'NONE', *, *, #1728, .F. ) ;
#47313=EDGE_CURVE ( 'NONE', #9420, #10431, #25803, .T. ) ;
#47320=ORIENTED_EDGE ( 'NONE', *, *, #32412, .T. ) ;
#47328=DIRECTION ( 'NONE',  ( 0.000000000000000000, 1.000000000000000000, -0.000000000000000000 ) ) ;
#47330=LINE ( 'NONE', #13794, #34678 ) ;
#47332=FACE_OUTER_BOUND ( 'NONE', #7544, .T. ) ;
#47334=FACE_OUTER_BOUND ( 'NONE', #28117, .T. ) ;
#47340=CARTESIAN_POINT ( 'NONE',  ( -13.92409385541305511, -10.10920654474410618, 80.49999999999998579 ) ) ;
#47344=ADVANCED_FACE ( 'NONE', ( #32561 ), #35529, .F. ) ;
#47356=ORIENTED_EDGE ( 'NONE', *, *, #37709, .F. ) ;
#47403=EDGE_CURVE ( 'NONE', #10587, #2752, #21096, .T. ) ;
#47499=DIRECTION ( 'NONE',  ( 0.000000000000000000, 0.000000000000000000, -1.000000000000000000 ) ) ;
#47534=CARTESIAN_POINT ( 'NONE',  ( -26.42409385541305511, -6.359206544744109735, 63.99999999999998579 ) ) ;
#47539=DIRECTION ( 'NONE',  ( 2.168404344971008375E-16, 0.000000000000000000, -1.000000000000000000 ) ) ;
#47543=AXIS2_PLACEMENT_3D ( 'NONE', #966, #12046, #46265 ) ;
#47560=DIRECTION ( 'NONE',  ( 0.000000000000000000, 0.000000000000000000, 1.000000000000000000 ) ) ;
#47613=ADVANCED_FACE ( 'NONE', ( #26890 ), #33759, .T. ) ;
#47622=EDGE_CURVE ( 'NONE', #3842, #27657, #36021, .T. ) ;
#47625=DIRECTION ( 'NONE',  ( 0.000000000000000000, 0.000000000000000000, 1.000000000000000000 ) ) ;
#47649=ORIENTED_EDGE ( 'NONE', *, *, #11237, .T. ) ;
#47657=CARTESIAN_POINT ( 'NONE',  ( -27.42409385541305156, -15.80920654474410725, 47.99999999999997868 ) ) ;
#47668=CARTESIAN_POINT ( 'NONE',  ( -27.42409385541305511, -27.10920654474410796, 78.99999999999998579 ) ) ;
#47675=ORIENTED_EDGE ( 'NONE', *, *, #1037, .F. ) ;
#47687=EDGE_CURVE ( 'NONE', #5074, #8993, #15554, .T. ) ;
#47709=AXIS2_PLACEMENT_3D ( 'NONE', #43563, #12781, #31980 ) ;
#47712=DIRECTION ( 'NONE',  ( 0.000000000000000000, 0.000000000000000000, 1.000000000000000000 ) ) ;
#47719=ORIENTED_EDGE ( 'NONE', *, *, #47687, .T. ) ;
#47724=CARTESIAN_POINT ( 'NONE',  ( -16.94712425470457973, -14.65920654474411045, 47.99999999999998579 ) ) ;
#47728=EDGE_CURVE ( 'NONE', #11393, #24008, #13531, .T. ) ;
#47736=ORIENTED_EDGE ( 'NONE', *, *, #13537, .F. ) ;
#47767=CARTESIAN_POINT ( 'NONE',  ( -4.424093855413053333, -25.10920654474410441, 63.99999999999998579 ) ) ;
#47805=AXIS2_PLACEMENT_3D ( 'NONE', #18358, #41029, #29699 ) ;
#47821=AXIS2_PLACEMENT_3D ( 'NONE', #39215, #1543, #47094 ) ;
#47841=ORIENTED_EDGE ( 'NONE', *, *, #41004, .T. ) ;
#47843=CIRCLE ( 'NONE', #38373, 0.5000000000000004441 ) ;
#47924=DIRECTION ( 'NONE',  ( 0.000000000000000000, 0.000000000000000000, 1.000000000000000000 ) ) ;
#47948=CARTESIAN_POINT ( 'NONE',  ( -35.32409385541306079, -6.359206544744109735, 48.79999999999998295 ) ) ;
#47949=VECTOR ( 'NONE', #10317, 1000.000000000000000 ) ;
#47955=VECTOR ( 'NONE', #30661, 1000.000000000000000 ) ;
#47956=ORIENTED_EDGE ( 'NONE', *, *, #12735, .T. ) ;
#47957=EDGE_LOOP ( 'NONE', ( #44900, #9842, #24079, #47649 ) ) ;
#47969=VECTOR ( 'NONE', #41583, 1000.000000000000000 ) ;
#47974=CARTESIAN_POINT ( 'NONE',  ( -27.42409385541305511, -27.10920654474410796, 81.99999999999998579 ) ) ;
#48019=ORIENTED_EDGE ( 'NONE', *, *, #14215, .T. ) ;
#48037=AXIS2_PLACEMENT_3D ( 'NONE', #41065, #7345, #7585 ) ;
#48040=DIRECTION ( 'NONE',  ( -0.000000000000000000, 1.000000000000000000, -0.000000000000000000 ) ) ;
#48048=AXIS2_PLACEMENT_3D ( 'NONE', #33059, #21034, #13625 ) ;
#48088=EDGE_CURVE ( 'NONE', #45046, #34652, #17907, .T. ) ;
#48114=AXIS2_PLACEMENT_3D ( 'NONE', #23097, #42042, #46471 ) ;
#48125=ORIENTED_EDGE ( 'NONE', *, *, #32461, .T. ) ;
#48140=DIRECTION ( 'NONE',  ( 1.927470528863119295E-16, 0.000000000000000000, -1.000000000000000000 ) ) ;
#48142=EDGE_CURVE ( 'NONE', #37234, #27864, #6100, .T. ) ;
#48161=DIRECTION ( 'NONE',  ( -1.000000000000000000, 0.000000000000000000, 0.000000000000000000 ) ) ;
#48219=CARTESIAN_POINT ( 'NONE',  ( -28.42409385541305511, -6.359206544744109735, 47.99999999999997868 ) ) ;
#48283=VERTEX_POINT ( 'NONE', #14656 ) ;
#48307=PLANE ( 'NONE',  #40768 ) ;
#48317=VERTEX_POINT ( 'NONE', #21010 ) ;
#48329=DIRECTION ( 'NONE',  ( 1.927470528863119542E-16, 0.000000000000000000, -1.000000000000000000 ) ) ;
#48362=ORIENTED_EDGE ( 'NONE', *, *, #35322, .F. ) ;
#48394=CARTESIAN_POINT ( 'NONE',  ( -46.92409385541305511, -17.80920654474410370, 62.75000000000000000 ) ) ;
#48405=CIRCLE ( 'NONE', #32660, 1.500000000000001332 ) ;
#48411=DIRECTION ( 'NONE',  ( -0.000000000000000000, -1.000000000000000000, -0.000000000000000000 ) ) ;
#48428=DIRECTION ( 'NONE',  ( 1.000000000000000000, 0.000000000000000000, -2.406186529621654018E-16 ) ) ;
#48450=ORIENTED_EDGE ( 'NONE', *, *, #6911, .F. ) ;
#48469=VERTEX_POINT ( 'NONE', #40675 ) ;
#48472=VECTOR ( 'NONE', #6643, 1000.000000000000000 ) ;
#48492=ADVANCED_FACE ( 'NONE', ( #3745 ), #48307, .T. ) ;
#48493=VERTEX_POINT ( 'NONE', #21973 ) ;
#48546=EDGE_CURVE ( 'NONE', #34669, #14458, #1253, .T. ) ;
#48569=MANIFOLD_SOLID_BREP ( 'Stock-MAS-175-1', #11842 ) ;
#48586=EDGE_LOOP ( 'NONE', ( #9348, #15117, #30947, #47058, #14751 ) ) ;
#48588=CARTESIAN_POINT ( 'NONE',  ( -7.424093855413048892, -25.10920654474410441, 77.00000000000000000 ) ) ;
#48597=VERTEX_POINT ( 'NONE', #1026 ) ;
#48610=EDGE_CURVE ( 'NONE', #29613, #42423, #27365, .T. ) ;
#48634=CARTESIAN_POINT ( 'NONE',  ( -28.42409385541305511, -25.10920654474410441, 52.99999999999997158 ) ) ;
#48670=EDGE_LOOP ( 'NONE', ( #1659, #45284 ) ) ;
#48702=LINE ( 'NONE', #12188, #36122 ) ;
ENDSEC;
END-ISO-10303-21;
